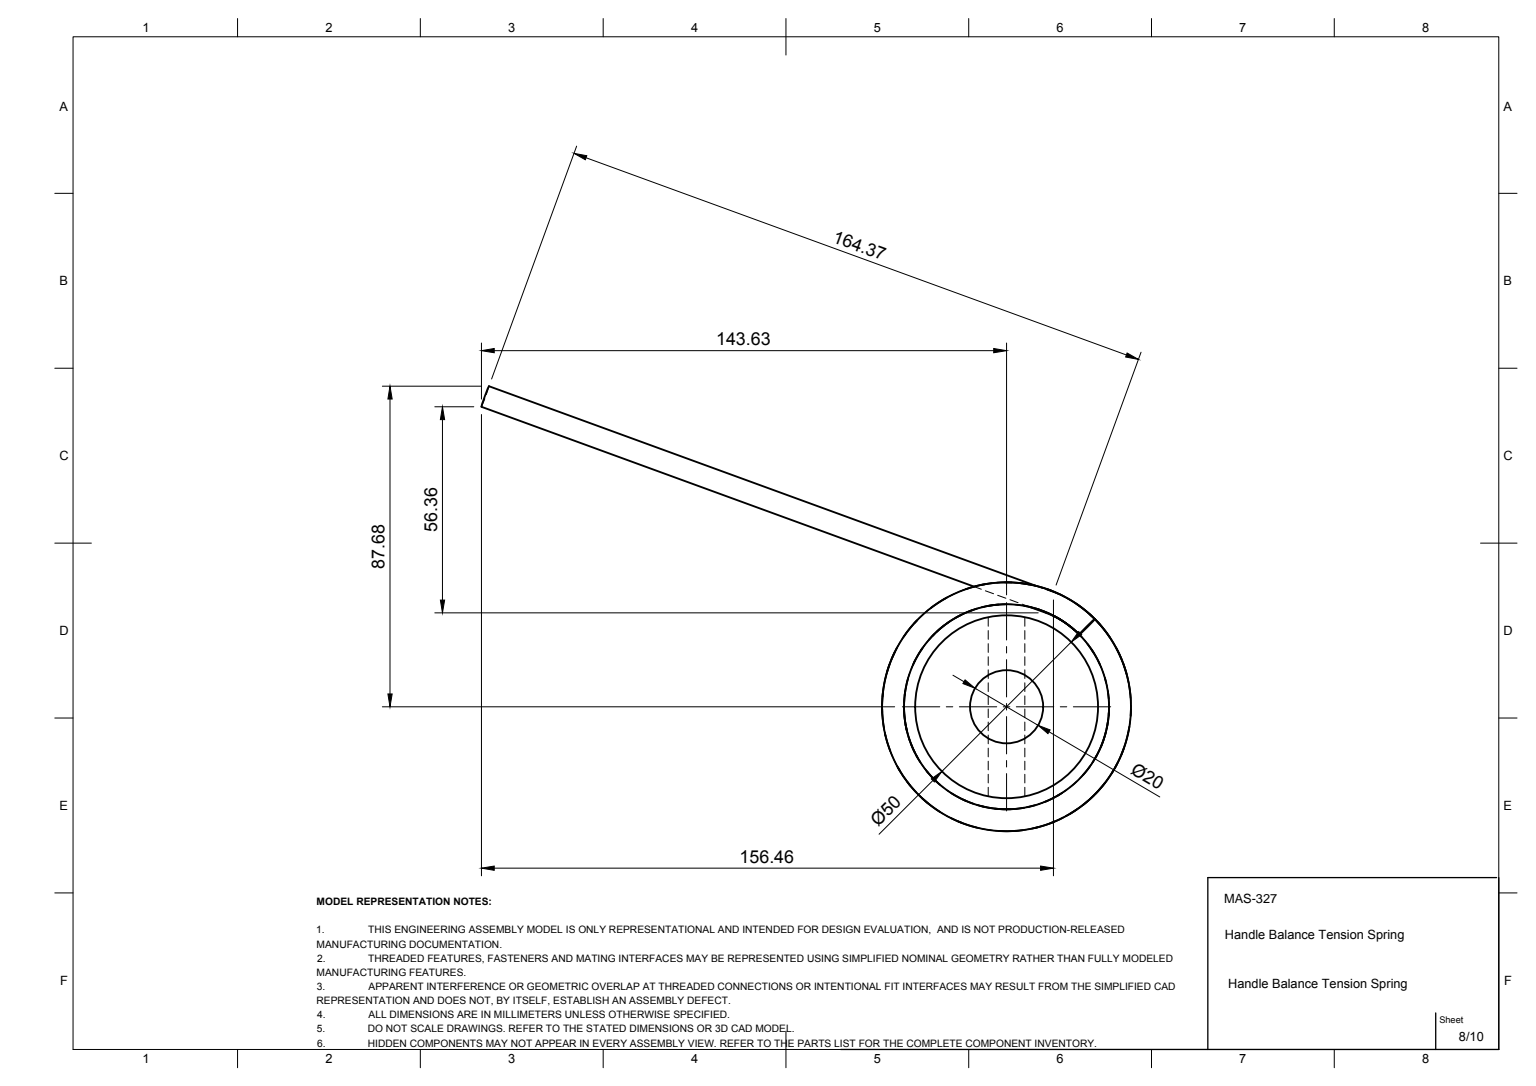
ISO-10303-21;
HEADER;
FILE_DESCRIPTION (('STEP AP214'),
    '1' );
FILE_NAME ('Handle Balance Tension Spring.step',
    '2026-10-06T22:16:42',
    ( '' ),
    ( '' ),
    'SwSTEP 2.0',
    'SolidWorks 2025',
    '' );
FILE_SCHEMA (( 'AUTOMOTIVE_DESIGN' ));
ENDSEC;

DATA;
#5=CARTESIAN_POINT ( 'NONE',  ( 71.26135857449716582, 118.5824631887579272, 4.723566274445706092 ) ) ;
#17=CARTESIAN_POINT ( 'NONE',  ( 22.10153057061799231, 100.9866247252079745, 1.346821830042071566 ) ) ;
#19=CARTESIAN_POINT ( 'NONE',  ( 8.829984022807513711, 121.7968051057545580, 16.14860047415989541 ) ) ;
#30=CARTESIAN_POINT ( 'NONE',  ( 39.19820123626366382, 154.0079489008930693, -4.284297094604833767 ) ) ;
#39=CARTESIAN_POINT ( 'NONE',  ( 43.64334309031418968, 148.0990856179656419, -3.057864931601543823 ) ) ;
#44=CARTESIAN_POINT ( 'NONE',  ( 72.37431012622080573, 137.3510900982057308, 5.986230922049878167 ) ) ;
#53=CARTESIAN_POINT ( 'NONE',  ( 58.35211712195835076, 96.24552883246097679, -7.224606741634919338 ) ) ;
#59=CARTESIAN_POINT ( 'NONE',  ( 77.24268685965694203, 120.2105100216710696, 12.57728155048203433 ) ) ;
#61=CARTESIAN_POINT ( 'NONE',  ( 40.36503175183082703, 91.91162403226272204, -5.481956346182379924 ) ) ;
#81=CARTESIAN_POINT ( 'NONE',  ( 15.47577296012077142, 113.4559151263126040, 0.9141320964044082897 ) ) ;
#87=CARTESIAN_POINT ( 'NONE',  ( 16.50170782505827560, 141.4403336307199197, 3.843654360456687513 ) ) ;
#89=CARTESIAN_POINT ( 'NONE',  ( 29.72792815944318789, 144.7825833525567134, 3.370790685444458479 ) ) ;
#101=CARTESIAN_POINT ( 'NONE',  ( 60.64192606672164487, 149.1585417170215067, -15.56126092485307488 ) ) ;
#109=CARTESIAN_POINT ( 'NONE',  ( 20.88913110926514705, 146.0313881486468119, 3.053432864643822686 ) ) ;
#116=CARTESIAN_POINT ( 'NONE',  ( 14.84555331229717012, 122.4588817147608637, 1.271029365619425144 ) ) ;
#128=CARTESIAN_POINT ( 'NONE',  ( 43.27907770151751521, 148.0257240122537610, -16.07737750751418915 ) ) ;
#140=CARTESIAN_POINT ( 'NONE',  ( 61.83586340360074018, 91.21788411573329824, -1.307985002297802568 ) ) ;
#146=CARTESIAN_POINT ( 'NONE',  ( 9.468627745026951814, 113.0646104733145592, 1.862908727141013854 ) ) ;
#148=CARTESIAN_POINT ( 'NONE',  ( 57.39747520560054284, 144.1616143014069280, -9.486357586414486676 ) ) ;
#154=CARTESIAN_POINT ( 'NONE',  ( 19.03178791447554374, 95.58698510358173905, 9.200771007679692914 ) ) ;
#163=CARTESIAN_POINT ( 'NONE',  ( 16.16443657470430750, 128.5343009702184816, -4.486436360144259616 ) ) ;
#170=DIRECTION ( 'NONE',  ( 1.000000000000000000, 0.000000000000000000, -0.000000000000000000 ) ) ;
#171=CARTESIAN_POINT ( 'NONE',  ( 19.13088699441526686, 95.37848931739559077, 15.19637875606281341 ) ) ;
#173=CARTESIAN_POINT ( 'NONE',  ( 63.17392202723403472, 139.5086487405075673, -1.196242060499778992 ) ) ;
#185=CARTESIAN_POINT ( 'NONE',  ( 14.84555331229717012, 122.4588817147608637, 1.271029365619425144 ) ) ;
#189=CARTESIAN_POINT ( 'NONE',  ( 9.953047844039691228, 128.4882722429139505, 3.367556520687803090 ) ) ;
#190=CARTESIAN_POINT ( 'NONE',  ( 17.20459894546975832, 108.5405110446994001, 1.704077971530460811 ) ) ;
#201=CARTESIAN_POINT ( 'NONE',  ( 44.01981256007524479, 154.0451711359460774, -9.132611258894215212 ) ) ;
#212=CARTESIAN_POINT ( 'NONE',  ( 23.00888394656308122, 147.7027690514567837, -4.855972970016076751 ) ) ;
#219=CARTESIAN_POINT ( 'NONE',  ( 26.43292637418678126, 142.8198486544370098, 2.223537717183381002 ) ) ;
#230=CARTESIAN_POINT ( 'NONE',  ( 33.52710748945926866, 93.34978808121778115, 14.79936193957723312 ) ) ;
#235=CARTESIAN_POINT ( 'NONE',  ( 48.01153233465171866, 95.41220631508043937, 33.88560042642480852 ) ) ;
#245=CARTESIAN_POINT ( 'NONE',  ( 40.94072057685551869, 85.65469043817564909, -0.5939954219232065347 ) ) ;
#251=CARTESIAN_POINT ( 'NONE',  ( 22.46358530849972723, 92.52609567587644790, 8.053519324161520387 ) ) ;
#253=CARTESIAN_POINT ( 'NONE',  ( 60.80507725967250821, 98.03074643439879310, -7.343579217248467295 ) ) ;
#262=CARTESIAN_POINT ( 'NONE',  ( 10.61900875472251649, 108.8314319666055212, -5.279948415675857376 ) ) ;
#272=CARTESIAN_POINT ( 'NONE',  ( 46.66836841558743032, 147.8683539324387368, -2.938892455568735240 ) ) ;
#282=CARTESIAN_POINT ( 'NONE',  ( 68.61421220432494295, 108.2796574941523886, 7.137043325852385323 ) ) ;
#287=ORIENTED_EDGE ( 'NONE', *, *, #12395, .T. ) ;
#301=CARTESIAN_POINT ( 'NONE',  ( 58.57740969237692497, 96.29577388269515836, -1.228997851713355072 ) ) ;
#306=CARTESIAN_POINT ( 'NONE',  ( 15.75986397150585816, 99.18880659646561071, -5.637120474378671808 ) ) ;
#307=CARTESIAN_POINT ( 'NONE',  ( 40.57367117788501787, 91.81261228707245436, 0.5136478283763052932 ) ) ;
#326=CARTESIAN_POINT ( 'NONE',  ( 77.24268685965694203, 120.2105100216710696, 12.57728155048203433 ) ) ;
#332=CARTESIAN_POINT ( 'NONE',  ( 31.11878897118147336, 145.5659923423516773, -4.562434011626001151 ) ) ;
#333=EDGE_CURVE ( 'NONE', #19172, #12901, #10944, .T. ) ;
#334=PRESENTATION_STYLE_ASSIGNMENT (( #15435 ) ) ;
#346=CARTESIAN_POINT ( 'NONE',  ( 42.37836782381873491, 91.71465960395167372, 14.44224817795539373 ) ) ;
#351=CARTESIAN_POINT ( 'NONE',  ( 48.01127559942236900, 95.41215390922535278, 34.53968432338328398 ) ) ;
#353=MANIFOLD_SOLID_BREP ( 'Cut-Extrude12', #11261 ) ;
#359=CARTESIAN_POINT ( 'NONE',  ( 62.34613790317991544, 148.1570561279473850, 11.50573666851796339 ) ) ;
#366=CARTESIAN_POINT ( 'NONE',  ( 8.869018199820361659, 117.4101421016551967, 9.005765870029716069 ) ) ;
#368=CARTESIAN_POINT ( 'NONE',  ( 50.21395344324809429, 147.1711500555979626, 4.203964687196366512 ) ) ;
#374=CARTESIAN_POINT ( 'NONE',  ( 29.43094928344231320, 88.48265962617873015, 0.7917390523231137012 ) ) ;
#382=CARTESIAN_POINT ( 'NONE',  ( 71.13433436327568415, 121.9840874124550965, -8.414894741535439593 ) ) ;
#387=ORIENTED_EDGE ( 'NONE', *, *, #9191, .T. ) ;
#392=CARTESIAN_POINT ( 'NONE',  ( 53.81137604271221164, 145.8702381773545653, 5.351212940250758443 ) ) ;
#395=EDGE_LOOP ( 'NONE', ( #15244, #20080, #9642, #2712 ) ) ;
#409=CARTESIAN_POINT ( 'NONE',  ( 31.65106594408818097, 87.52743543124788062, 20.71565594656193454 ) ) ;
#413=CARTESIAN_POINT ( 'NONE',  ( 21.78317867943344766, 93.15162560046918827, 9.081842247139665147 ) ) ;
#414=CARTESIAN_POINT ( 'NONE',  ( 67.15412698936957270, 134.4792784496449087, 12.06138812558265805 ) ) ;
#423=CARTESIAN_POINT ( 'NONE',  ( 10.57123148683770175, 130.5870355106474108, -10.56118268746274325 ) ) ;
#434=CARTESIAN_POINT ( 'NONE',  ( 68.80033453084351436, 142.5431462587704061, -3.212652714419679700 ) ) ;
#440=CARTESIAN_POINT ( 'NONE',  ( 58.08784223975295902, 95.98046199469133910, 5.794885020722011504 ) ) ;
#450=CARTESIAN_POINT ( 'NONE',  ( 32.23767430054685690, 145.5917660130465379, 17.43780275515692679 ) ) ;
#460=VERTEX_POINT ( 'NONE', #20827 ) ;
#462=CARTESIAN_POINT ( 'NONE',  ( 52.46025766099742071, 152.8098426157893925, 11.14871012209260748 ) ) ;
#467=CARTESIAN_POINT ( 'NONE',  ( 40.02721236285810136, 85.80382532021769748, 0.4343372985580923329 ) ) ;
#469=CARTESIAN_POINT ( 'NONE',  ( 41.25620118372704326, 148.0523446076144580, 3.846850258842608117 ) ) ;
#477=CARTESIAN_POINT ( 'NONE',  ( 20.22230697948889500, 94.36241449208007737, 1.148710122009321211 ) ) ;
#481=CARTESIAN_POINT ( 'NONE',  ( 63.55746018358933469, 147.2895578332197033, -9.446739241148069510 ) ) ;
#494=CARTESIAN_POINT ( 'NONE',  ( 77.13564277734779751, 118.5067815986552375, -14.37074460762677397 ) ) ;
#512=CARTESIAN_POINT ( 'NONE',  ( 26.48090744323847190, 142.7828511622217889, -4.776412194962503577 ) ) ;
#518=CARTESIAN_POINT ( 'NONE',  ( 9.616596702810701558, 112.3753283828585694, -5.161025107254184618 ) ) ;
#519=CARTESIAN_POINT ( 'NONE',  ( 65.09246388851926213, 137.4469437283422906, 4.918530982704383270 ) ) ;
#527=CARTESIAN_POINT ( 'NONE',  ( 42.70556344282044137, 85.75549003223034106, 1.343541076088082376 ) ) ;
#534=CARTESIAN_POINT ( 'NONE',  ( 42.21854335081802390, 85.68333463812091111, 14.36287948008016890 ) ) ;
#540=CARTESIAN_POINT ( 'NONE',  ( 15.53544334784188585, 126.6048195653137469, 15.43757839183889224 ) ) ;
#551=CARTESIAN_POINT ( 'NONE',  ( 63.85057544308668298, 100.9084186779620609, 13.48995955233852229 ) ) ;
#553=CARTESIAN_POINT ( 'NONE',  ( 43.66339603962469340, 144.9006758593374968, 29.24238570022250627 ) ) ;
#556=CARTESIAN_POINT ( 'NONE',  ( 47.56746500088171814, 95.32565373869623215, 32.14446507322556101 ) ) ;
#563=CARTESIAN_POINT ( 'NONE',  ( 26.28242620001017471, 89.94675250444232972, 6.906269859504051922 ) ) ;
#569=CARTESIAN_POINT ( 'NONE',  ( 74.85601106972485752, 107.3429126181175661, -0.9942341299615756745 ) ) ;
#571=CARTESIAN_POINT ( 'NONE',  ( 32.47916914626341622, 146.0660553311768979, 3.489959554161691013 ) ) ;
#580=CARTESIAN_POINT ( 'NONE',  ( 51.60797029699607918, 86.77139250312444574, -6.946567135388369785 ) ) ;
#600=CARTESIAN_POINT ( 'NONE',  ( 19.41497643977705323, 135.2012136132025546, 3.803670830490076149 ) ) ;
#603=CYLINDRICAL_SURFACE ( 'NONE', #15728, 10.00000000000000888 ) ;
#621=CARTESIAN_POINT ( 'NONE',  ( 54.90439719837324617, 94.24896709312837118, 12.93774216356182372 ) ) ;
#627=CARTESIAN_POINT ( 'NONE',  ( 26.87026879109711786, 150.0197496251087728, 11.30891725959585159 ) ) ;
#628=CARTESIAN_POINT ( 'NONE',  ( 68.77576173894735234, 108.4446202281264249, 13.13264940013829296 ) ) ;
#639=CARTESIAN_POINT ( 'NONE',  ( 41.12929731208597417, 154.0090796829547912, -2.227802639778228233 ) ) ;
#648=CARTESIAN_POINT ( 'NONE',  ( 9.231363607564425422, 125.4582397780895633, 16.26765482522027639 ) ) ;
#654=CARTESIAN_POINT ( 'NONE',  ( 46.21245884545565019, 91.80782910428004584, 13.29499484581607582 ) ) ;
#664=CARTESIAN_POINT ( 'NONE',  ( 55.97020510223934764, 144.8627979930266463, -1.553355716038981038 ) ) ;
#676=CARTESIAN_POINT ( 'NONE',  ( 13.60337824163328513, 137.5875211305428252, 8.692014997358331385 ) ) ;
#685=CARTESIAN_POINT ( 'NONE',  ( 70.03002323795641360, 111.8333997399938511, 5.989792257250448060 ) ) ;
#691=CARTESIAN_POINT ( 'NONE',  ( 61.61057083318216598, 91.16763906547615193, -7.303593892219363504 ) ) ;
#703=CARTESIAN_POINT ( 'NONE',  ( 69.71972837475884432, 98.49221204361529658, -7.660766391518695428 ) ) ;
#710=CARTESIAN_POINT ( 'NONE',  ( 43.31828379119179573, 154.0590585871367750, -16.15632009132952973 ) ) ;
#731=CARTESIAN_POINT ( 'NONE',  ( 18.61283035262889385, 105.6058852300018032, 7.580709131559767222 ) ) ;
#738=CARTESIAN_POINT ( 'NONE',  ( 38.34086628137072239, 86.07498427433979771, 8.486398261126511855 ) ) ;
#739=CARTESIAN_POINT ( 'NONE',  ( 16.97565887011968400, 109.0741130153051444, 8.727962422049884594 ) ) ;
#746=CARTESIAN_POINT ( 'NONE',  ( 31.96084264191244273, 87.59053552682176758, 1.700516636338098797 ) ) ;
#754=CARTESIAN_POINT ( 'NONE',  ( 29.59780345622613851, 88.32329120701308511, 6.787350155335245994 ) ) ;
#760=CARTESIAN_POINT ( 'NONE',  ( 70.16915148685765757, 112.0176666281686977, 11.98539833154344691 ) ) ;
#774=CARTESIAN_POINT ( 'NONE',  ( 32.71008791447857789, 146.0719641954536883, -2.505641559509553140 ) ) ;
#776=CARTESIAN_POINT ( 'NONE',  ( 45.52055293674428071, 144.7823678009017954, 38.54804764342389944 ) ) ;
#781=DIRECTION ( 'NONE',  ( 0.9387810623359076345, 0.3426822732243071656, 0.03548206049944094970 ) ) ;
#785=CARTESIAN_POINT ( 'NONE',  ( 51.15470623622070434, 86.57325545146775880, 6.072769092256255163 ) ) ;
#793=CARTESIAN_POINT ( 'NONE',  ( 67.98812442775457043, 106.8157236907426153, -0.7957547315468347371 ) ) ;
#800=CARTESIAN_POINT ( 'NONE',  ( 75.16956835342354282, 131.6452004531123805, 5.196376467030073165 ) ) ;
#809=CARTESIAN_POINT ( 'NONE',  ( 75.85495621331871519, 129.5603373922052697, -8.732165470513974626 ) ) ;
#815=CARTESIAN_POINT ( 'NONE',  ( 15.58850788081759475, 140.2644050767460442, -10.20415289822252980 ) ) ;
#836=CARTESIAN_POINT ( 'NONE',  ( 29.49905557571407044, 144.7517438296894738, 9.366394860000250233 ) ) ;
#842=CARTESIAN_POINT ( 'NONE',  ( 18.20936163119166196, 143.5026679720446907, 2.934308097026923967 ) ) ;
#843=CARTESIAN_POINT ( 'NONE',  ( 65.44800906011916197, 136.9904114405718758, 11.94221925691594777 ) ) ;
#844=CARTESIAN_POINT ( 'NONE',  ( 20.98687704487253569, 141.7792436784441747, -11.00219731500033049 ) ) ;
#853=CARTESIAN_POINT ( 'NONE',  ( 9.783399875253829592, 127.8057224500684015, -3.656374068424393275 ) ) ;
#855=CARTESIAN_POINT ( 'NONE',  ( 70.26356658872128946, 140.6255928306487704, 11.86290872716119615 ) ) ;
#861=CARTESIAN_POINT ( 'NONE',  ( 10.61292492956169475, 108.6005711365770026, 0.7156557588857267449 ) ) ;
#869=CARTESIAN_POINT ( 'NONE',  ( 43.17520790721623314, 91.62706341066298421, 13.41396976009479403 ) ) ;
#878=CARTESIAN_POINT ( 'NONE',  ( 14.99696000743431235, 117.4761687382565327, -3.934212988072375516 ) ) ;
#891=CARTESIAN_POINT ( 'NONE',  ( 54.37136329154349568, 152.2862128563062072, 3.215626235130811583 ) ) ;
#898=CARTESIAN_POINT ( 'NONE',  ( 39.35338560254503903, 91.94623120232463975, 14.56122079753911081 ) ) ;
#904=CARTESIAN_POINT ( 'NONE',  ( 62.84376099716368458, 92.00366499689042143, 13.64888190966157566 ) ) ;
#915=CARTESIAN_POINT ( 'NONE',  ( 15.75986397150585816, 99.18880659646561071, -5.637120474378671808 ) ) ;
#925=ORIENTED_EDGE ( 'NONE', *, *, #19064, .F. ) ;
#940=CARTESIAN_POINT ( 'NONE',  ( 40.78231060393920870, 91.71360054188218669, 6.509252002934985626 ) ) ;
#946=CARTESIAN_POINT ( 'NONE',  ( 57.14511974427749408, 88.72838517433189054, 6.862995836283489304 ) ) ;
#948=CARTESIAN_POINT ( 'NONE',  ( 16.70103016558074316, 129.9804388327498827, 16.57432765154378629 ) ) ;
#949=CARTESIAN_POINT ( 'NONE',  ( 26.28921445626723852, 149.7786157371718616, -3.732453678475698311 ) ) ;
#959=CARTESIAN_POINT ( 'NONE',  ( 47.07528247981900904, 85.99676402675389397, -5.799316066731655006 ) ) ;
#961=CARTESIAN_POINT ( 'NONE',  ( 31.47436479266152531, 87.67613096727390598, 14.72005176623422606 ) ) ;
#968=CARTESIAN_POINT ( 'NONE',  ( 75.01029411920679024, 107.5147569559006655, 5.001370044594233732 ) ) ;
#974=CARTESIAN_POINT ( 'NONE',  ( 70.54646159239726444, 126.3605644061445901, 18.41388650843374464 ) ) ;
#982=ORIENTED_EDGE ( 'NONE', *, *, #5579, .F. ) ;
#987=CARTESIAN_POINT ( 'NONE',  ( 68.32201692705490359, 132.1587870917933003, -0.8393580998851425390 ) ) ;
#990=CARTESIAN_POINT ( 'NONE',  ( 46.98099381664906815, 144.5901365555967004, 37.25520735466820810 ) ) ;
#996=CARTESIAN_POINT ( 'NONE',  ( 23.17700876947760591, 147.8092992330439586, -3.851376987104358829 ) ) ;
#1003=CARTESIAN_POINT ( 'NONE',  ( 73.37616494982036386, 135.8902282719419077, 4.049127002338204662 ) ) ;
#1012=CARTESIAN_POINT ( 'NONE',  ( 33.52710748945926866, 93.34978808121778115, 14.79936193957723312 ) ) ;
#1019=CARTESIAN_POINT ( 'NONE',  ( 71.03835150376274044, 100.2492380157770526, 6.267546321443639989 ) ) ;
#1028=CARTESIAN_POINT ( 'NONE',  ( 57.94507594753278568, 150.7106492751291569, -2.660852849641732298 ) ) ;
#1036=ADVANCED_FACE ( 'NONE', ( #2390 ), #7256, .F. ) ;
#1052=CARTESIAN_POINT ( 'NONE',  ( 34.49559591455799534, 146.8750064778945728, 2.580435534661669195 ) ) ;
#1055=DIRECTION ( 'NONE',  ( -1.000000000000000000, 0.000000000000000000, 0.000000000000000000 ) ) ;
#1058=CARTESIAN_POINT ( 'NONE',  ( 54.54805624998882507, 152.1374805055981199, -2.779977617235711129 ) ) ;
#1060=CARTESIAN_POINT ( 'NONE',  ( 43.85786119575681852, 148.0137586191354444, -9.053472026759274982 ) ) ;
#1062=CARTESIAN_POINT ( 'NONE',  ( 23.67598417054553295, 91.65793073385727041, -5.994147020910363999 ) ) ;
#1072=CARTESIAN_POINT ( 'NONE',  ( 8.922311181598237440, 122.0085103898528018, 10.15299703236346573 ) ) ;
#1075=CARTESIAN_POINT ( 'NONE',  ( 72.33162239183086228, 137.5781058455011703, 11.98183203572534872 ) ) ;
#1080=CARTESIAN_POINT ( 'NONE',  ( 43.59077634914400079, 154.2158251336064723, 2.858602931426994953 ) ) ;
#1086=CARTESIAN_POINT ( 'NONE',  ( 58.78870511939484800, 143.3781512503299780, 17.58070913143554748 ) ) ;
#1091=PLANE ( 'NONE',  #19799 ) ;
#1097=CARTESIAN_POINT ( 'NONE',  ( 37.89917375590665927, 147.5588116854153498, -9.291614562240097186 ) ) ;
#1098=CARTESIAN_POINT ( 'NONE',  ( 43.66945230930459587, 144.9005013971865594, 39.17809732472422013 ) ) ;
#1104=CARTESIAN_POINT ( 'NONE',  ( 23.67598417054553295, 91.65793073385727041, -5.994147020910363999 ) ) ;
#1112=CARTESIAN_POINT ( 'NONE',  ( 41.39294982251618649, 154.1830292177732531, 16.78735015533800734 ) ) ;
#1119=CARTESIAN_POINT ( 'NONE',  ( 25.64412274706724304, 97.69032544021251852, 15.15625305551708202 ) ) ;
#1127=CARTESIAN_POINT ( 'NONE',  ( 40.90832812944997698, 154.0758954209757121, 3.767805038447253452 ) ) ;
#1128=CARTESIAN_POINT ( 'NONE',  ( 40.50225576765475921, 95.03178743630938641, 38.54804764342390655 ) ) ;
#1136=CARTESIAN_POINT ( 'NONE',  ( 69.83118287335672392, 141.1824132108841638, 4.838974892866481525 ) ) ;
#1161=CARTESIAN_POINT ( 'NONE',  ( 39.55749537675153960, 91.83829536962669238, 20.55682687220188143 ) ) ;
#1167=CARTESIAN_POINT ( 'NONE',  ( 47.47886434171987702, 153.8471147930492862, -3.017879606865911502 ) ) ;
#1168=CARTESIAN_POINT ( 'NONE',  ( 68.06566224877710169, 132.6756899087416457, -7.863043133634088910 ) ) ;
#1176=CARTESIAN_POINT ( 'NONE',  ( 56.11190468687431832, 151.4478768383145280, 5.272225788895710252 ) ) ;
#1181=EDGE_CURVE ( 'NONE', #11596, #5848, #13724, .T. ) ;
#1185=CARTESIAN_POINT ( 'NONE',  ( 9.585575214713108139, 112.1464265272871188, 0.8345760063739874335 ) ) ;
#1191=CARTESIAN_POINT ( 'NONE',  ( 66.16974147772015158, 135.9983230778657344, -9.010293137571032673 ) ) ;
#1200=CARTESIAN_POINT ( 'NONE',  ( 48.12388674207330297, 92.25590008057444891, 8.208355790051324874 ) ) ;
#1204=CARTESIAN_POINT ( 'NONE',  ( 47.85046472749336743, 144.4343633168767269, 32.91075569967801329 ) ) ;
#1220=CARTESIAN_POINT ( 'NONE',  ( 10.76517401744387215, 131.6399553617083029, 15.47769843104460463 ) ) ;
#1223=CARTESIAN_POINT ( 'NONE',  ( 9.504183449854689769, 113.2927979568517571, -4.132695447411913747 ) ) ;
#1226=CARTESIAN_POINT ( 'NONE',  ( 14.85320491933239317, 121.4429315054255909, 16.22795414098078126 ) ) ;
#1230=CARTESIAN_POINT ( 'NONE',  ( 15.00983914341701997, 123.2415857317943448, 2.299110145932334426 ) ) ;
#1232=CARTESIAN_POINT ( 'NONE',  ( 65.27013532398795803, 145.9152199903044504, 11.62486143609835310 ) ) ;
#1243=CARTESIAN_POINT ( 'NONE',  ( 26.90790578767411390, 150.1165885900122987, 3.291480155758420345 ) ) ;
#1269=CARTESIAN_POINT ( 'NONE',  ( 69.69253243162556544, 129.2828754355126648, 18.29472124897268159 ) ) ;
#1276=CARTESIAN_POINT ( 'NONE',  ( 63.41425016244589585, 92.41789933959738335, 6.624947895572852019 ) ) ;
#1277=CARTESIAN_POINT ( 'NONE',  ( 69.05514009256096131, 130.5101840208823205, -14.76775785107876082 ) ) ;
#1294=CARTESIAN_POINT ( 'NONE',  ( 26.67903320394502131, 150.0857490671680807, 9.287084330314211655 ) ) ;
#1301=CARTESIAN_POINT ( 'NONE',  ( 59.92122946415073415, 142.4742691614619332, -9.367183195626855863 ) ) ;
#1311=CARTESIAN_POINT ( 'NONE',  ( 33.24893159794274311, 146.2783277815063059, 4.518043653832040540 ) ) ;
#1321=CARTESIAN_POINT ( 'NONE',  ( 46.60148787037231699, 85.86292235506145687, 7.220022382731924537 ) ) ;
#1328=CARTESIAN_POINT ( 'NONE',  ( 63.06653971011325410, 92.06373373134326243, 19.64449301269484849 ) ) ;
#1329=CIRCLE ( 'NONE', #8736, 24.99999999999999289 ) ;
#1332=CARTESIAN_POINT ( 'NONE',  ( 15.69291839309778958, 99.40984958608130739, -11.63272432674803802 ) ) ;
#1336=CARTESIAN_POINT ( 'NONE',  ( 44.86974823489592978, 148.0457227541334362, 10.98970740178311090 ) ) ;
#1341=CARTESIAN_POINT ( 'NONE',  ( 17.20459894546975832, 108.5405110446994001, 1.704077971530460811 ) ) ;
#1345=CARTESIAN_POINT ( 'NONE',  ( 41.71169011715027608, 94.93878194014966709, 29.37128083581765381 ) ) ;
#1355=CARTESIAN_POINT ( 'NONE',  ( 26.13368487350976110, 90.12329638092472806, 0.9106621812756837686 ) ) ;
#1379=CARTESIAN_POINT ( 'NONE',  ( 26.70363248220801466, 142.8423586596025245, -10.77201286955609127 ) ) ;
#1385=CARTESIAN_POINT ( 'NONE',  ( 16.30372524420941716, 141.3216567370616019, 9.839263250375132941 ) ) ;
#1388=CARTESIAN_POINT ( 'NONE',  ( 40.25662930883660806, 147.8909896968035014, -16.19631701608006580 ) ) ;
#1405=CARTESIAN_POINT ( 'NONE',  ( 62.21295035458982881, 148.3457431455455549, 17.50134052088148096 ) ) ;
#1412=CARTESIAN_POINT ( 'NONE',  ( 24.63684302007652249, 148.6959638282970957, 4.200683933265449532 ) ) ;
#1413=CARTESIAN_POINT ( 'NONE',  ( 69.04633063039527485, 130.7408809369782716, -8.772150750671475095 ) ) ;
#1423=CARTESIAN_POINT ( 'NONE',  ( 15.29689364450883815, 124.6620785063593786, 10.35143954082134954 ) ) ;
#1433=CARTESIAN_POINT ( 'NONE',  ( 67.39040179371399120, 143.9404232637865562, 4.720051584306741432 ) ) ;
#1442=CARTESIAN_POINT ( 'NONE',  ( 21.21153947156776809, 146.4065673692475400, 16.07276909216647454 ) ) ;
#1446=CARTESIAN_POINT ( 'NONE',  ( 13.64837572802379562, 102.4646860582014796, -11.51360178106338594 ) ) ;
#1454=CARTESIAN_POINT ( 'NONE',  ( 63.07923660420441792, 139.7192868340247571, 4.799362114056002326 ) ) ;
#1466=CARTESIAN_POINT ( 'NONE',  ( 40.90832812944997698, 154.0758954209757121, 3.767805038447253452 ) ) ;
#1472=CARTESIAN_POINT ( 'NONE',  ( 61.61057083318216598, 91.16763906547615193, -7.303593892219363504 ) ) ;
#1492=CARTESIAN_POINT ( 'NONE',  ( 19.04663372520828801, 134.9227921665808765, 15.79488502079956547 ) ) ;
#1498=CARTESIAN_POINT ( 'NONE',  ( 55.94180145820917716, 151.6039095241057453, 11.26783467880839140 ) ) ;
#1499=CARTESIAN_POINT ( 'NONE',  ( 47.44511438772692458, 147.6747606579048409, -1.910614883896327054 ) ) ;
#1517=CARTESIAN_POINT ( 'NONE',  ( 70.82039710638956365, 99.80338443054456832, 19.28708432993385102 ) ) ;
#1522=CARTESIAN_POINT ( 'NONE',  ( 59.50342836137831171, 89.99885106877826502, 7.772197353298202493 ) ) ;
#1523=CARTESIAN_POINT ( 'NONE',  ( 55.20039838223064521, 94.47806301326188816, -0.08174959847185196693 ) ) ;
#1532=CARTESIAN_POINT ( 'NONE',  ( 71.12409474721032154, 120.5409021055102841, -0.3630727742139398528 ) ) ;
#1544=CARTESIAN_POINT ( 'NONE',  ( 47.30009524607925897, 85.94413156685014599, 0.1962900075584997628 ) ) ;
#1551=CARTESIAN_POINT ( 'NONE',  ( 22.89857099655110062, 139.5608133708311982, -4.966967973427480310 ) ) ;
#1554=CARTESIAN_POINT ( 'NONE',  ( 17.52322149637394233, 97.17389352242535949, -4.727774211004094340 ) ) ;
#1564=CARTESIAN_POINT ( 'NONE',  ( 25.21830160582964453, 141.7844325674071229, 10.15653385063274428 ) ) ;
#1567=CARTESIAN_POINT ( 'NONE',  ( 15.97061701817242785, 140.8453463817331794, 16.82122940411608170 ) ) ;
#1576=CARTESIAN_POINT ( 'NONE',  ( 53.71239221804358976, 87.38980250447106357, 6.982120393166105998 ) ) ;
#1583=CARTESIAN_POINT ( 'NONE',  ( 40.73010619540765020, 85.74955863377461185, -6.589596535617429751 ) ) ;
#1585=CARTESIAN_POINT ( 'NONE',  ( 26.70363248220801466, 142.8423586596025245, -10.77201286955609127 ) ) ;
#1589=CARTESIAN_POINT ( 'NONE',  ( 62.62098228421420032, 91.94359626243755201, 7.653270806628301948 ) ) ;
#1597=CARTESIAN_POINT ( 'NONE',  ( 57.03263806925237844, 95.34629841206742640, 19.84245794357962822 ) ) ;
#1604=CARTESIAN_POINT ( 'NONE',  ( 76.40658810299491677, 127.4365358892444959, 12.33923360994393903 ) ) ;
#1605=CARTESIAN_POINT ( 'NONE',  ( 54.97053026609068382, 94.45704024927961484, -6.077358488390353308 ) ) ;
#1623=CARTESIAN_POINT ( 'NONE',  ( 63.63589212299756070, 92.48244826560708987, 12.62055557379543203 ) ) ;
#1628=CARTESIAN_POINT ( 'NONE',  ( 67.48508721674359379, 143.7297851702464015, -1.275552590249036777 ) ) ;
#1629=CARTESIAN_POINT ( 'NONE',  ( 49.55020742284296631, 92.47612394764220767, 0.1565338505643876776 ) ) ;
#1641=CARTESIAN_POINT ( 'NONE',  ( 54.44380493464903736, 94.21656919670213881, 0.9465279732350617703 ) ) ;
#1653=CARTESIAN_POINT ( 'NONE',  ( 73.72238702602700755, 135.0318370961144296, 5.077453337991364002 ) ) ;
#1659=CARTESIAN_POINT ( 'NONE',  ( 66.44170838958859804, 135.7440291252205213, 4.009006963233090026 ) ) ;
#1673=CARTESIAN_POINT ( 'NONE',  ( 70.94289844336020678, 123.7826807253454575, 5.513563639855703080 ) ) ;
#1687=CARTESIAN_POINT ( 'NONE',  ( 75.87089013534350102, 129.7906142932847331, -2.736556584054479657 ) ) ;
#1694=CARTESIAN_POINT ( 'NONE',  ( 69.71972837475884432, 98.49221204361529658, -7.660766391518695428 ) ) ;
#1698=CARTESIAN_POINT ( 'NONE',  ( 16.33471683235446292, 110.7640000046674089, -5.200637885961103102 ) ) ;
#1704=CARTESIAN_POINT ( 'NONE',  ( 71.86557814238962294, 101.4853659568252766, -7.779689512009451136 ) ) ;
#1712=CARTESIAN_POINT ( 'NONE',  ( 71.19430100617981338, 118.9508470517051535, -8.295922056425867552 ) ) ;
#1721=CARTESIAN_POINT ( 'NONE',  ( 9.231363607564425422, 125.4582397780895633, 16.26765482522027639 ) ) ;
#1723=CARTESIAN_POINT ( 'NONE',  ( 24.98902006629997175, 141.4916631675600343, -2.862956674147950409 ) ) ;
#1736=CARTESIAN_POINT ( 'NONE',  ( 71.19881468907274780, 122.2058620619881566, -2.419290889312981641 ) ) ;
#1742=CARTESIAN_POINT ( 'NONE',  ( 42.70556344282044137, 85.75549003223034106, 1.343541076088082376 ) ) ;
#1743=CARTESIAN_POINT ( 'NONE',  ( 62.66823040046688931, 140.1266048904901993, -2.224326160187301227 ) ) ;
#1751=DIRECTION ( 'NONE',  ( 0.000000000000000000, 0.000000000000000000, 1.000000000000000000 ) ) ;
#1754=CARTESIAN_POINT ( 'NONE',  ( 29.68407903333335085, 144.6596297928226988, 11.33750686376150085 ) ) ;
#1763=CARTESIAN_POINT ( 'NONE',  ( 9.468627745026951814, 113.0646104733145592, 1.862908727141013854 ) ) ;
#1770=CARTESIAN_POINT ( 'NONE',  ( 18.91286941000743838, 105.1068529970173699, 0.5568269029779387980 ) ) ;
#1783=CARTESIAN_POINT ( 'NONE',  ( 53.64127281404707048, 146.0262708631457542, 11.34682183016344403 ) ) ;
#1792=CARTESIAN_POINT ( 'NONE',  ( 39.03606557573836255, 144.5896687849443651, 31.16068397573688387 ) ) ;
#1795=ORIENTED_EDGE ( 'NONE', *, *, #13768, .T. ) ;
#1798=CARTESIAN_POINT ( 'NONE',  ( 64.81014823317600815, 93.40725510594978687, -1.427111354441281899 ) ) ;
#1803=CARTESIAN_POINT ( 'NONE',  ( 73.32203938827501588, 103.9946350594383517, -0.8753108214479579097 ) ) ;
#1805=CARTESIAN_POINT ( 'NONE',  ( 49.02192908010439254, 147.4586317741252799, -9.843465619175002956 ) ) ;
#1811=CARTESIAN_POINT ( 'NONE',  ( 42.00398509169406935, 85.76881261499585207, 8.367275628961508005 ) ) ;
#1820=CARTESIAN_POINT ( 'NONE',  ( 68.03731475862628031, 132.9047928164914367, -1.867435455408581912 ) ) ;
#1827=CARTESIAN_POINT ( 'NONE',  ( 28.07864021081662287, 89.10199518432737875, 14.83897397183228861 ) ) ;
#1829=CARTESIAN_POINT ( 'NONE',  ( 70.19721620597543676, 127.0927327670264475, -7.624900598222268400 ) ) ;
#1846=CARTESIAN_POINT ( 'NONE',  ( 50.34320592624661828, 92.59351467088818310, -0.8717445255428065698 ) ) ;
#1850=CARTESIAN_POINT ( 'NONE',  ( 20.25093610150840107, 136.5556286039603435, -4.129180435126924564 ) ) ;
#1853=VERTEX_POINT ( 'NONE', #14705 ) ;
#1854=DIRECTION ( 'NONE',  ( 0.000000000000000000, 0.000000000000000000, 1.000000000000000000 ) ) ;
#1860=CARTESIAN_POINT ( 'NONE',  ( 39.64555921537804295, 153.8934876517313342, -16.27550955686750456 ) ) ;
#1869=CARTESIAN_POINT ( 'NONE',  ( 23.42018083028975184, 147.9700754799198705, 17.16443675223517573 ) ) ;
#1875=CARTESIAN_POINT ( 'NONE',  ( 70.23874406963963679, 127.5525917602273012, 4.366313592093098883 ) ) ;
#1885=CARTESIAN_POINT ( 'NONE',  ( 17.81206540393426252, 132.5069038242342003, 16.68302557436956945 ) ) ;
#1891=CARTESIAN_POINT ( 'NONE',  ( 41.71002329038685730, 144.8752540357612020, 29.37189892749851694 ) ) ;
#1896=CARTESIAN_POINT ( 'NONE',  ( 42.21854335081802390, 85.68333463812091111, 14.36287948008016890 ) ) ;
#1901=CARTESIAN_POINT ( 'NONE',  ( 20.98687704487253569, 141.7792436784441747, -11.00219731500033049 ) ) ;
#1903=CARTESIAN_POINT ( 'NONE',  ( 46.60148787037231699, 85.86292235506145687, 7.220022382731924537 ) ) ;
#1911=CARTESIAN_POINT ( 'NONE',  ( 9.468627745026951814, 113.0646104733145592, 1.862908727141013854 ) ) ;
#1921=CARTESIAN_POINT ( 'NONE',  ( 55.29376081731632553, 145.2908078538121401, -2.581636314160848489 ) ) ;
#1927=ORIENTED_EDGE ( 'NONE', *, *, #17355, .T. ) ;
#1932=CARTESIAN_POINT ( 'NONE',  ( 50.52618006956270591, 153.2232370340747138, -15.91843667049845834 ) ) ;
#1944=CARTESIAN_POINT ( 'NONE',  ( 18.86674891209848326, 143.9013856721611546, -11.04182128657428485 ) ) ;
#1951=CARTESIAN_POINT ( 'NONE',  ( 16.02160000510927418, 128.3529272436884128, 1.509170735004851549 ) ) ;
#1955=CARTESIAN_POINT ( 'NONE',  ( 30.08091612619420729, 88.20954595054467973, -6.232194961517499188 ) ) ;
#1956=CARTESIAN_POINT ( 'NONE',  ( 14.81332417359726783, 119.6334487847019403, -4.843746996953559147 ) ) ;
#1967=CARTESIAN_POINT ( 'NONE',  ( 20.91795382191701336, 137.2581800298614212, 10.90446256675174297 ) ) ;
#1977=CARTESIAN_POINT ( 'NONE',  ( 45.29500579500201951, 154.0643053174194961, 10.91066218119221709 ) ) ;
#1983=CARTESIAN_POINT ( 'NONE',  ( 14.73513546934961482, 119.4163655414939740, 1.151864106104608432 ) ) ;
#1984=SURFACE_SIDE_STYLE ('',( #20397 ) ) ;
#1996=CARTESIAN_POINT ( 'NONE',  ( 31.57890723221301599, 145.5991046824261446, -16.55366158474257432 ) ) ;
#2002=CARTESIAN_POINT ( 'NONE',  ( 44.62651314315545648, 94.95745790197152303, 38.95396702123348831 ) ) ;
#2007=ORIENTED_EDGE ( 'NONE', *, *, #6812, .F. ) ;
#2010=CARTESIAN_POINT ( 'NONE',  ( 32.07966263401961982, 152.4337125855422528, -4.522337938825778281 ) ) ;
#2017=CARTESIAN_POINT ( 'NONE',  ( 17.14282613681034917, 97.48634091255654255, 8.291567264837656381 ) ) ;
#2019=CARTESIAN_POINT ( 'NONE',  ( 15.50679444821833819, 113.6848169819070193, -5.081469017220888063 ) ) ;
#2027=CARTESIAN_POINT ( 'NONE',  ( 40.73010619540765020, 85.74955863377461185, -6.589596535617429751 ) ) ;
#2034=CARTESIAN_POINT ( 'NONE',  ( 41.15066532084431827, 91.76888749123396849, -6.510040445920065366 ) ) ;
#2044=CARTESIAN_POINT ( 'NONE',  ( 21.19424684193554143, 137.6478987072957807, 3.922641511544080917 ) ) ;
#2064=CARTESIAN_POINT ( 'NONE',  ( 29.98029990418277180, 151.1550010424932111, 23.43402463578956585 ) ) ;
#2068=CARTESIAN_POINT ( 'NONE',  ( 64.59149290518072917, 93.33317027722591774, -7.422718449586769296 ) ) ;
#2070=CARTESIAN_POINT ( 'NONE',  ( 61.33076419740685736, 141.3451534613812441, 11.70407797152743079 ) ) ;
#2078=CARTESIAN_POINT ( 'NONE',  ( 73.43285993012185031, 135.4320224564883688, -7.942088354107054826 ) ) ;
#2087=CARTESIAN_POINT ( 'NONE',  ( 14.48810111090402941, 100.9784058478479523, 15.43442115621699529 ) ) ;
#2093=CARTESIAN_POINT ( 'NONE',  ( 41.03523200113699687, 148.1191603456353789, 9.842457937073838536 ) ) ;
#2101=CARTESIAN_POINT ( 'NONE',  ( 58.92189266798492042, 143.1894642327317513, 11.58510527907202992 ) ) ;
#2103=CARTESIAN_POINT ( 'NONE',  ( 45.22414464412956647, 144.8093836198929694, 29.72396354041403299 ) ) ;
#2115=CARTESIAN_POINT ( 'NONE',  ( 12.43312601512511151, 135.2277911470865490, 16.60371454366222466 ) ) ;
#2121=CARTESIAN_POINT ( 'NONE',  ( 30.24639091383375700, 151.6717570033048048, 3.410403464249057492 ) ) ;
#2123=CARTESIAN_POINT ( 'NONE',  ( 16.97565887011968400, 109.0741130153051444, 8.727962422049884594 ) ) ;
#2130=CARTESIAN_POINT ( 'NONE',  ( 17.73005198514846725, 142.9879744078657779, -4.089424278207452801 ) ) ;
#2132=CARTESIAN_POINT ( 'NONE',  ( 20.22230697948889500, 94.36241449208007737, 1.148710122009321211 ) ) ;
#2137=CARTESIAN_POINT ( 'NONE',  ( 40.73010619540765020, 85.74955863377461185, -6.589596535617429751 ) ) ;
#2149=CARTESIAN_POINT ( 'NONE',  ( 75.83902229129397199, 129.3300604911257778, -14.72777435697347137 ) ) ;
#2165=CARTESIAN_POINT ( 'NONE',  ( 70.48772827241290884, 113.2068808858050630, -2.062176545857650201 ) ) ;
#2169=CARTESIAN_POINT ( 'NONE',  ( 30.38027039762175718, 151.3010018550503446, 11.44158087452429129 ) ) ;
#2170=CARTESIAN_POINT ( 'NONE',  ( 63.07923660420441792, 139.7192868340247571, 4.799362114056002326 ) ) ;
#2180=CARTESIAN_POINT ( 'NONE',  ( 29.91082003397629663, 88.36561978549612206, -12.22780263974880022 ) ) ;
#2193=CARTESIAN_POINT ( 'NONE',  ( 62.34613790317991544, 148.1570561279473850, 11.50573666851796339 ) ) ;
#2200=CARTESIAN_POINT ( 'NONE',  ( 17.32321720400341292, 131.7349665092470730, 8.652027877775747555 ) ) ;
#2210=CARTESIAN_POINT ( 'NONE',  ( 51.29519266978688563, 92.95216133272363379, 14.08499220319455780 ) ) ;
#2216=CARTESIAN_POINT ( 'NONE',  ( 43.01140435219951286, 94.90707761860558378, 39.21067981925356349 ) ) ;
#2223=CARTESIAN_POINT ( 'NONE',  ( 61.24245875951225315, 90.83725678726602837, 5.715745788549559059 ) ) ;
#2228=CARTESIAN_POINT ( 'NONE',  ( 29.43094928344231320, 88.48265962617873015, 0.7917390523231137012 ) ) ;
#2231=CARTESIAN_POINT ( 'NONE',  ( 69.25106277675128297, 109.5764507715396832, -0.9149236002526208722 ) ) ;
#2237=CARTESIAN_POINT ( 'NONE',  ( 76.04618105687035268, 128.8835079444423286, -1.708432735116285350 ) ) ;
#2247=CARTESIAN_POINT ( 'NONE',  ( 76.04618105687035268, 128.8835079444423286, -1.708432735116285350 ) ) ;
#2248=FACE_OUTER_BOUND ( 'NONE', #9607, .T. ) ;
#2253=CARTESIAN_POINT ( 'NONE',  ( 15.21076168709227616, 115.6846582791190201, 9.994193321846964295 ) ) ;
#2269=CARTESIAN_POINT ( 'NONE',  ( 50.02529374262071826, 147.3041493969045064, 10.19957357710909207 ) ) ;
#2273=CARTESIAN_POINT ( 'NONE',  ( 9.248697603757472407, 114.7582530722838356, 9.914954709382596931 ) ) ;
#2274=CARTESIAN_POINT ( 'NONE',  ( 25.64412274706724304, 97.69032544021251852, 15.15625305551708202 ) ) ;
#2283=CARTESIAN_POINT ( 'NONE',  ( 46.37776046713125311, 85.92026137128108587, 1.224418530371263580 ) ) ;
#2286=CARTESIAN_POINT ( 'NONE',  ( 26.66797635711824199, 149.9459070286683868, 17.30505193804556185 ) ) ;
#2292=CARTESIAN_POINT ( 'NONE',  ( 9.976645104453018220, 110.9295780357170571, 15.79146183154218619 ) ) ;
#2298=CARTESIAN_POINT ( 'NONE',  ( 47.04142330690687857, 147.8988775214238842, 10.08059930640748902 ) ) ;
#2311=CARTESIAN_POINT ( 'NONE',  ( 24.98902006629997175, 141.4916631675600343, -2.862956674147950409 ) ) ;
#2313=CARTESIAN_POINT ( 'NONE',  ( 46.31438439993811329, 144.6890179153603242, 30.44285285587857715 ) ) ;
#2318=CARTESIAN_POINT ( 'NONE',  ( 45.51857396895002239, 95.03161353365992170, 38.54896506029344749 ) ) ;
#2322=ADVANCED_FACE ( 'NONE', ( #14541 ), #13705, .T. ) ;
#2325=CARTESIAN_POINT ( 'NONE',  ( 69.47322557110069852, 98.06143112153284846, 5.358778726746561638 ) ) ;
#2333=CARTESIAN_POINT ( 'NONE',  ( 66.10898071834657230, 103.7292514542787245, 6.347102411281516865 ) ) ;
#2341=CARTESIAN_POINT ( 'NONE',  ( 77.19215121279506775, 118.0176990621192203, -1.351406188750652992 ) ) ;
#2354=CARTESIAN_POINT ( 'NONE',  ( 60.49690154327523572, 149.3382625450468311, -9.565656633516235630 ) ) ;
#2360=CARTESIAN_POINT ( 'NONE',  ( 32.54106024366770811, 152.4163610972421452, -16.51355214031335805 ) ) ;
#2381=CARTESIAN_POINT ( 'NONE',  ( 68.16012629694054681, 106.9699110742356396, 5.199846382127304878 ) ) ;
#2384=AXIS2_PLACEMENT_3D ( 'NONE', #2478, #21008, #4241 ) ;
#2388=CARTESIAN_POINT ( 'NONE',  ( 74.62708615766334219, 133.0342049366344384, -8.851289726714327344 ) ) ;
#2389=CARTESIAN_POINT ( 'NONE',  ( 20.99626426110969390, 137.5292218135913913, 9.918250401459649979 ) ) ;
#2390=FACE_OUTER_BOUND ( 'NONE', #12530, .T. ) ;
#2398=CARTESIAN_POINT ( 'NONE',  ( 9.127117681521182746, 124.1904119534442401, -3.775300622140596030 ) ) ;
#2401=CARTESIAN_POINT ( 'NONE',  ( 9.231363607564425422, 125.4582397780895633, 16.26765482522027639 ) ) ;
#2403=CARTESIAN_POINT ( 'NONE',  ( 0.000000000000000000, 0.000000000000000000, 0.000000000000000000 ) ) ;
#2407=CARTESIAN_POINT ( 'NONE',  ( 77.31131846045057898, 118.9338434746808844, -2.379532457331845485 ) ) ;
#2412=CARTESIAN_POINT ( 'NONE',  ( 14.73996261871784341, 120.6514404024884755, 15.19984638209844441 ) ) ;
#2422=CARTESIAN_POINT ( 'NONE',  ( 70.19721620597543676, 127.0927327670264475, -7.624900598222268400 ) ) ;
#2435=CARTESIAN_POINT ( 'NONE',  ( 29.59780345622613851, 88.32329120701308511, 6.787350155335245994 ) ) ;
#2441=CARTESIAN_POINT ( 'NONE',  ( 70.84063976188440392, 115.3547488198113200, -1.153064885589385025 ) ) ;
#2449=CARTESIAN_POINT ( 'NONE',  ( 45.29500579500201951, 154.0643053174194961, 10.91066218119221709 ) ) ;
#2459=CARTESIAN_POINT ( 'NONE',  ( 44.41273964558330789, 85.70220254879866673, -6.708519844216274564 ) ) ;
#2465=CARTESIAN_POINT ( 'NONE',  ( 57.55288598684787615, 89.00415807515548750, -6.156345639627279986 ) ) ;
#2467=DIRECTION ( 'NONE',  ( 0.000000000000000000, 0.000000000000000000, -1.000000000000000000 ) ) ;
#2478=CARTESIAN_POINT ( 'NONE',  ( 43.01140435219951996, 119.9070776186055838, -35.00000000000000000 ) ) ;
#2484=CARTESIAN_POINT ( 'NONE',  ( 71.26135857449716582, 118.5824631887579272, 4.723566274445706092 ) ) ;
#2491=CARTESIAN_POINT ( 'NONE',  ( 73.32203938827501588, 103.9946350594383517, -0.8753108214479579097 ) ) ;
#2492=CARTESIAN_POINT ( 'NONE',  ( 69.68673170630326297, 129.0522134326295145, 12.29911014595921692 ) ) ;
#2502=CARTESIAN_POINT ( 'NONE',  ( 76.87285023715404009, 124.3600315475450486, -0.5611826874715375446 ) ) ;
#2504=CARTESIAN_POINT ( 'NONE',  ( 12.43312601512511151, 135.2277911470865490, 16.60371454366222466 ) ) ;
#2510=CARTESIAN_POINT ( 'NONE',  ( 9.433072040199128594, 112.8364229897773470, 7.858512901693939234 ) ) ;
#2516=CARTESIAN_POINT ( 'NONE',  ( 21.79768317403592803, 101.2052074350461339, 14.36631359211887649 ) ) ;
#2530=CARTESIAN_POINT ( 'NONE',  ( 20.44379504597808861, 136.6827000062168338, -10.12478428749056469 ) ) ;
#2532=CARTESIAN_POINT ( 'NONE',  ( 44.63189717924443300, 144.8563245053103401, 38.95199156105033467 ) ) ;
#2537=CARTESIAN_POINT ( 'NONE',  ( 44.41273964558330789, 85.70220254879866673, -6.708519844216274564 ) ) ;
#2543=CARTESIAN_POINT ( 'NONE',  ( 47.27474595639033339, 153.9548969447091906, 2.977729283044022957 ) ) ;
#2550=CARTESIAN_POINT ( 'NONE',  ( 58.43892221570314405, 143.5117748958429047, 4.561220828673259398 ) ) ;
#2557=CARTESIAN_POINT ( 'NONE',  ( 68.29446192123552350, 96.82662215664792882, 13.41040346623746515 ) ) ;
#2558=CARTESIAN_POINT ( 'NONE',  ( 38.67087568172628664, 95.28607559046729136, 36.71405245301004783 ) ) ;
#2567=CARTESIAN_POINT ( 'NONE',  ( 23.23160898551418185, 147.7622765488190453, -10.85157364460736140 ) ) ;
#2588=CARTESIAN_POINT ( 'NONE',  ( 29.27693512915957541, 95.18479568265063051, 6.985315079919499404 ) ) ;
#2594=CARTESIAN_POINT ( 'NONE',  ( 11.67247064774405452, 106.1322524520788875, 1.624861436118421043 ) ) ;
#2595=CARTESIAN_POINT ( 'NONE',  ( 32.21091799184858218, 93.94358800413606048, -12.14875741943239085 ) ) ;
#2596=CARTESIAN_POINT ( 'NONE',  ( 10.42839491720816625, 130.4056617841633283, -4.565575592310756825 ) ) ;
#2607=CARTESIAN_POINT ( 'NONE',  ( 27.13677837140323490, 150.1474281128565167, -2.704124018797368301 ) ) ;
#2614=CARTESIAN_POINT ( 'NONE',  ( 13.37233465371036090, 102.6159639102351093, 7.501340520787425525 ) ) ;
#2620=CARTESIAN_POINT ( 'NONE',  ( 64.30534519084480394, 138.3942263399134447, -9.129458798097310535 ) ) ;
#2621=( NAMED_UNIT ( * ) PLANE_ANGLE_UNIT ( ) SI_UNIT ( $, .RADIAN. ) );
#2631=CARTESIAN_POINT ( 'NONE',  ( 65.16383128666855384, 137.2272505635282585, -1.077070130972596962 ) ) ;
#2633=CARTESIAN_POINT ( 'NONE',  ( 48.01156915178761864, 144.4019414068667686, 34.53828804502998651 ) ) ;
#2646=CARTESIAN_POINT ( 'NONE',  ( 32.75162935850930523, 152.6515011162663313, 2.501635869428501469 ) ) ;
#2652=CARTESIAN_POINT ( 'NONE',  ( 58.92189266798492042, 143.1894642327317513, 11.58510527907202992 ) ) ;
#2653=ORIENTED_EDGE ( 'NONE', *, *, #14566, .F. ) ;
#2659=CARTESIAN_POINT ( 'NONE',  ( 69.83118287335672392, 141.1824132108841638, 4.838974892866481525 ) ) ;
#2660=CARTESIAN_POINT ( 'NONE',  ( 41.70806931348493407, 94.93898644073527748, 39.04902473919937478 ) ) ;
#2670=CARTESIAN_POINT ( 'NONE',  ( 74.62708615766334219, 133.0342049366344384, -8.851289726714327344 ) ) ;
#2680=VERTEX_POINT ( 'NONE', #15549 ) ;
#2689=STYLED_ITEM ( 'NONE', ( #6670 ), #14549 ) ;
#2698=CARTESIAN_POINT ( 'NONE',  ( 62.38482844916680392, 99.30468409114129713, 12.58043553469319953 ) ) ;
#2701=CARTESIAN_POINT ( 'NONE',  ( 43.01140435219951996, 119.9070776186055838, -35.00000000000000000 ) ) ;
#2705=CARTESIAN_POINT ( 'NONE',  ( 25.52397925108762067, 90.47728371212039633, 7.934596195134201224 ) ) ;
#2707=CARTESIAN_POINT ( 'NONE',  ( 52.12662541604375122, 146.5080492276505311, -15.72009227599853531 ) ) ;
#2709=CARTESIAN_POINT ( 'NONE',  ( 32.98198692859195802, 152.6383102900375093, -3.493975233523312962 ) ) ;
#2712=ORIENTED_EDGE ( 'NONE', *, *, #19599, .F. ) ;
#2718=CARTESIAN_POINT ( 'NONE',  ( 17.52322149637394233, 97.17389352242535949, -4.727774211004094340 ) ) ;
#2722=CARTESIAN_POINT ( 'NONE',  ( 24.41145734808947054, 148.6458414325078081, 10.19629000755267434 ) ) ;
#2729=CARTESIAN_POINT ( 'NONE',  ( 66.97354912532109950, 95.34500505098478129, 5.477698430975745048 ) ) ;
#2735=CARTESIAN_POINT ( 'NONE',  ( 32.03768905382736421, 145.5187656067679711, 23.43402463578956585 ) ) ;
#2747=CARTESIAN_POINT ( 'NONE',  ( 26.96882349746146446, 96.81297435472995971, -11.91061488385382106 ) ) ;
#2755=CARTESIAN_POINT ( 'NONE',  ( 20.91437931538276374, 145.9617080342048894, -10.94665030085253044 ) ) ;
#2763=CARTESIAN_POINT ( 'NONE',  ( 59.95958160670890180, 90.07020311440788873, 19.76341270931769500 ) ) ;
#2778=CARTESIAN_POINT ( 'NONE',  ( 52.46025766099742071, 152.8098426157893925, 11.14871012209260748 ) ) ;
#2785=CARTESIAN_POINT ( 'NONE',  ( 10.91571581598819662, 131.8149664739095783, 9.482090752819161139 ) ) ;
#2811=CARTESIAN_POINT ( 'NONE',  ( 35.68099593698222094, 147.2217917141817907, 16.62841781073025871 ) ) ;
#2817=CARTESIAN_POINT ( 'NONE',  ( 8.927628897234525240, 116.7075971571176751, 1.981832035706394546 ) ) ;
#2818=CARTESIAN_POINT ( 'NONE',  ( 26.92635752117756098, 142.9018661569831750, -16.76761354414967542 ) ) ;
#2825=CARTESIAN_POINT ( 'NONE',  ( 23.23160898551418185, 147.7622765488190453, -10.85157364460736140 ) ) ;
#2830=( NAMED_UNIT ( * ) PLANE_ANGLE_UNIT ( ) SI_UNIT ( $, .RADIAN. ) );
#2834=CARTESIAN_POINT ( 'NONE',  ( 55.35048440753327981, 87.88826800209452017, -1.070088050731120344 ) ) ;
#2840=CARTESIAN_POINT ( 'NONE',  ( 71.17671054099098171, 117.3556635612232810, 18.77100214853170357 ) ) ;
#2849=CARTESIAN_POINT ( 'NONE',  ( 56.57648482392179545, 95.27494636639178793, 7.851242587554376762 ) ) ;
#2859=CARTESIAN_POINT ( 'NONE',  ( 69.71972837475884432, 98.49221204361529658, -7.660766391518695428 ) ) ;
#2867=CARTESIAN_POINT ( 'NONE',  ( 74.43934690056714487, 106.1333445020626129, 19.04903893889577660 ) ) ;
#2871=CARTESIAN_POINT ( 'NONE',  ( 77.09984031027478579, 117.8059907461747429, -7.347010041119995449 ) ) ;
#2883=CARTESIAN_POINT ( 'NONE',  ( 27.67177345608778793, 143.5689829720894011, 10.27550654291302479 ) ) ;
#2886=CARTESIAN_POINT ( 'NONE',  ( 51.78234217841457365, 152.9971814535558963, 4.124977536042813142 ) ) ;
#2899=CARTESIAN_POINT ( 'NONE',  ( 10.16827731527805767, 110.2528774685086574, 8.767718578943870966 ) ) ;
#2923=CARTESIAN_POINT ( 'NONE',  ( 29.27949416537561333, 144.5119445999418986, 23.32977622066093204 ) ) ;
#2928=CYLINDRICAL_SURFACE ( 'NONE', #11527, 4.999999999999997335 ) ;
#2929=CARTESIAN_POINT ( 'NONE',  ( 72.98789752971651978, 103.3738663174133023, 6.148623012889737005 ) ) ;
#2930=CARTESIAN_POINT ( 'NONE',  ( 69.30627838890079317, 109.9422389716749535, -13.93421298911417416 ) ) ;
#2943=CARTESIAN_POINT ( 'NONE',  ( 13.97286934428321103, 138.1879231288898495, 15.71574578848041881 ) ) ;
#2950=CARTESIAN_POINT ( 'NONE',  ( 15.78326802858598299, 112.2624592280589439, 21.86641499745291028 ) ) ;
#2961=CARTESIAN_POINT ( 'NONE',  ( 42.16380956469475194, 91.80013758078052888, 8.446644326836734606 ) ) ;
#2964=DIRECTION ( 'NONE',  ( -1.000000000000000000, 0.000000000000000000, 0.000000000000000000 ) ) ;
#2971=CARTESIAN_POINT ( 'NONE',  ( 75.80354157443048280, 110.0810758630161672, 5.910575721798123183 ) ) ;
#2979=CARTESIAN_POINT ( 'NONE',  ( 8.737656864016759783, 121.5850998216562431, 22.14420391595633220 ) ) ;
#2983=CARTESIAN_POINT ( 'NONE',  ( 69.52170837389681424, 98.37355370181180092, -13.65637406972050272 ) ) ;
#2986=CARTESIAN_POINT ( 'NONE',  ( 69.85845278386915425, 111.2786852186620621, 13.01367670771671747 ) ) ;
#2991=CARTESIAN_POINT ( 'NONE',  ( 31.84750084766683287, 94.01163676417708359, 0.8705387173494113506 ) ) ;
#2996=CARTESIAN_POINT ( 'NONE',  ( 39.24730198293589467, 95.19097405389743471, 30.90345582088290044 ) ) ;
#3007=CARTESIAN_POINT ( 'NONE',  ( 48.17517050666977241, 153.7480039124125994, 4.005852979123367241 ) ) ;
#3023=DIRECTION ( 'NONE',  ( 0.9387810623359078566, 0.3426822732243069436, 0.03548206049944095664 ) ) ;
#3031=CARTESIAN_POINT ( 'NONE',  ( 32.03768905382736421, 145.5187656067679711, 23.43402463578956585 ) ) ;
#3037=CARTESIAN_POINT ( 'NONE',  ( 15.97061701817242785, 140.8453463817331794, 16.82122940411608170 ) ) ;
#3038=CARTESIAN_POINT ( 'NONE',  ( 14.89151287784495281, 119.8505320279099209, -10.83935810001172229 ) ) ;
#3055=CARTESIAN_POINT ( 'NONE',  ( 52.27439898384277939, 152.9467924839493946, 17.14431721725165758 ) ) ;
#3062=CARTESIAN_POINT ( 'NONE',  ( 31.34884810169724645, 145.5825485123889109, -10.55804779818428862 ) ) ;
#3073=CARTESIAN_POINT ( 'NONE',  ( 65.57965399412842089, 103.1314161556117028, 7.375186511277089352 ) ) ;
#3085=CARTESIAN_POINT ( 'NONE',  ( 66.76198117565915879, 95.25264312590786631, -0.5179092472497510702 ) ) ;
#3093=CARTESIAN_POINT ( 'NONE',  ( 42.43310160994198554, 85.59785666124599857, 20.35848333119881914 ) ) ;
#3097=CARTESIAN_POINT ( 'NONE',  ( 27.13677837140323490, 150.1474281128565167, -2.704124018797368301 ) ) ;
#3100=CARTESIAN_POINT ( 'NONE',  ( 65.77248029998415291, 103.2585056976580091, 13.37079068582577435 ) ) ;
#3106=CARTESIAN_POINT ( 'NONE',  ( 51.84853669763433004, 93.12814091139611605, 7.061107544354192633 ) ) ;
#3108=CARTESIAN_POINT ( 'NONE',  ( 14.48810111090402941, 100.9784058478479523, 15.43442115621699529 ) ) ;
#3115=EDGE_LOOP ( 'NONE', ( #387, #5902 ) ) ;
#3118=CARTESIAN_POINT ( 'NONE',  ( 71.03835150376274044, 100.2492380157770526, 6.267546321443639989 ) ) ;
#3125=CARTESIAN_POINT ( 'NONE',  ( 75.10802748102119608, 108.0013139708956800, -8.018167963582932600 ) ) ;
#3143=CARTESIAN_POINT ( 'NONE',  ( 51.52566954327383542, 92.93877768781105431, 20.08059929855049219 ) ) ;
#3149=CARTESIAN_POINT ( 'NONE',  ( 52.46025766099742071, 152.8098426157893925, 11.14871012209260748 ) ) ;
#3150=CARTESIAN_POINT ( 'NONE',  ( 70.62278752756289180, 114.5844828164671441, -0.1247842873985126749 ) ) ;
#3170=CARTESIAN_POINT ( 'NONE',  ( 77.17837728419731036, 116.7372127726149245, 18.69201499742705153 ) ) ;
#3175=CARTESIAN_POINT ( 'NONE',  ( 70.43474449472395804, 99.54920534645194152, 7.295875980836476593 ) ) ;
#3176=CARTESIAN_POINT ( 'NONE',  ( 69.25106277675128297, 109.5764507715396832, -0.9149236002526208722 ) ) ;
#3187=CARTESIAN_POINT ( 'NONE',  ( 27.89715912807487186, 143.6191053679247602, 4.279900468622926724 ) ) ;
#3198=CARTESIAN_POINT ( 'NONE',  ( 71.03835150376274044, 100.2492380157770526, 6.267546321443639989 ) ) ;
#3205=CARTESIAN_POINT ( 'NONE',  ( 10.15219960346482431, 110.0225462658725490, 14.76332465322822074 ) ) ;
#3208=CARTESIAN_POINT ( 'NONE',  ( 29.26409511065843105, 88.64202804534433255, -5.203872050689020590 ) ) ;
#3216=CARTESIAN_POINT ( 'NONE',  ( 66.10898071834657230, 103.7292514542787245, 6.347102411281516865 ) ) ;
#3228=CARTESIAN_POINT ( 'NONE',  ( 50.92548328124963319, 86.60151408976496157, 0.07716523989554470442 ) ) ;
#3236=CARTESIAN_POINT ( 'NONE',  ( 73.40451243997107156, 135.6611253642151098, -1.946480675884423084 ) ) ;
#3239=CARTESIAN_POINT ( 'NONE',  ( 16.16443657470430750, 128.5343009702184816, -4.486436360144259616 ) ) ;
#3244=CARTESIAN_POINT ( 'NONE',  ( 53.88337135589062399, 152.3674195137575964, -9.803719146365084569 ) ) ;
#3254=CIRCLE ( 'NONE', #21207, 3.000000000000000444 ) ;
#3256=CARTESIAN_POINT ( 'NONE',  ( 18.01452421378985136, 106.6802099491036273, 21.62814552769798837 ) ) ;
#3261=FACE_OUTER_BOUND ( 'NONE', #9156, .T. ) ;
#3262=CARTESIAN_POINT ( 'NONE',  ( 22.01597290215339697, 101.2010103422484519, -4.648787059867797389 ) ) ;
#3279=CARTESIAN_POINT ( 'NONE',  ( 73.69864372527810303, 135.2613471474284097, 11.07306444099484466 ) ) ;
#3284=CARTESIAN_POINT ( 'NONE',  ( 61.89860894053757789, 148.3622700476249463, -1.513601781051955530 ) ) ;
#3286=CARTESIAN_POINT ( 'NONE',  ( 50.21395344324809429, 147.1711500555979626, 4.203964687196366512 ) ) ;
#3298=CARTESIAN_POINT ( 'NONE',  ( 21.19424684193554143, 137.6478987072957807, 3.922641511544080917 ) ) ;
#3309=CARTESIAN_POINT ( 'NONE',  ( 17.14282613681034917, 97.48634091255654255, 8.291567264837656381 ) ) ;
#3317=CARTESIAN_POINT ( 'NONE',  ( 52.31916092102454741, 146.6125112339981627, 3.294994845742023948 ) ) ;
#3327=CARTESIAN_POINT ( 'NONE',  ( 68.29827362630597065, 132.3882971431532383, 5.156253003121209488 ) ) ;
#3335=CARTESIAN_POINT ( 'NONE',  ( 38.51811260612901577, 144.5002972345523631, 36.42795439419948877 ) ) ;
#3340=CARTESIAN_POINT ( 'NONE',  ( 28.65042173108665935, 151.0721679115347911, -4.641026357035400451 ) ) ;
#3346=CARTESIAN_POINT ( 'NONE',  ( 50.33192209904863290, 153.3481575868430014, -9.922832680162505525 ) ) ;
#3349=CARTESIAN_POINT ( 'NONE',  ( 34.72595348466361287, 146.8618156516888291, -3.415175568290148345 ) ) ;
#3356=CARTESIAN_POINT ( 'NONE',  ( 76.20123706073158587, 111.5182621349952257, -8.137091297256032973 ) ) ;
#3367=CARTESIAN_POINT ( 'NONE',  ( 57.86150831142030171, 95.93494642397840266, -0.2007220744356660869 ) ) ;
#3373=FACE_BOUND ( 'NONE', #21625, .T. ) ;
#3374=CARTESIAN_POINT ( 'NONE',  ( 74.27779736592162863, 105.9683817680885056, 13.05343286460986363 ) ) ;
#3375=CARTESIAN_POINT ( 'NONE',  ( 15.79683473163509966, 126.9851207307152521, 3.446356185820485418 ) ) ;
#3393=CARTESIAN_POINT ( 'NONE',  ( 67.29571637068438861, 144.1510613573267108, 10.71565575886252297 ) ) ;
#3398=CARTESIAN_POINT ( 'NONE',  ( 70.84804472268019992, 100.1183116193850964, 0.2719452077637916076 ) ) ;
#3399=CARTESIAN_POINT ( 'NONE',  ( 18.57470074671828542, 105.8336742703428257, 1.585105279193314010 ) ) ;
#3411=CARTESIAN_POINT ( 'NONE',  ( 43.01140435219951996, 119.9070776186055838, 50.00000000000002842 ) ) ;
#3414=CARTESIAN_POINT ( 'NONE',  ( 27.04509496028088478, 143.0549882411833380, 11.23409068567602098 ) ) ;
#3426=CARTESIAN_POINT ( 'NONE',  ( 35.69068542950036260, 86.46542255174357194, 7.577194441455407770 ) ) ;
#3433=CARTESIAN_POINT ( 'NONE',  ( 70.48772827241290884, 113.2068808858050630, -2.062176545857650201 ) ) ;
#3443=CARTESIAN_POINT ( 'NONE',  ( 69.85845278386915425, 111.2786852186620621, 13.01367670771671747 ) ) ;
#3457=CARTESIAN_POINT ( 'NONE',  ( 12.61881386508366809, 104.1535352963828984, 15.55354899318430739 ) ) ;
#3461=DIRECTION ( 'NONE',  ( 1.000000000000000000, 0.000000000000000000, 0.000000000000000000 ) ) ;
#3463=CARTESIAN_POINT ( 'NONE',  ( 69.83118287335672392, 141.1824132108841638, 4.838974892866481525 ) ) ;
#3471=CARTESIAN_POINT ( 'NONE',  ( 59.50342836137831171, 89.99885106877826502, 7.772197353298202493 ) ) ;
#3481=CARTESIAN_POINT ( 'NONE',  ( 32.38101408406643600, 93.78751416920769657, -6.153149741203968404 ) ) ;
#3487=CARTESIAN_POINT ( 'NONE',  ( 77.07719282571002850, 116.5297446719512209, 12.69640610750513865 ) ) ;
#3490=CARTESIAN_POINT ( 'NONE',  ( 17.65293208513390866, 132.0582047407114885, -3.339186312533837242 ) ) ;
#3491=EDGE_CURVE ( 'NONE', #1853, #4221, #21002, .T. ) ;
#3505=CARTESIAN_POINT ( 'NONE',  ( 9.955767346236717330, 110.6995739201198887, 21.78706596723887756 ) ) ;
#3509=CARTESIAN_POINT ( 'NONE',  ( 41.12929731208597417, 154.0090796829547912, -2.227802639778228233 ) ) ;
#3510=CARTESIAN_POINT ( 'NONE',  ( 70.21798013780751546, 127.3226622636268672, -1.629293503064584536 ) ) ;
#3520=CARTESIAN_POINT ( 'NONE',  ( 15.69291839309778958, 99.40984958608130739, -11.63272432674803802 ) ) ;
#3530=CARTESIAN_POINT ( 'NONE',  ( 18.14018356548558941, 143.3940520581896862, 16.92415443696469879 ) ) ;
#3536=CARTESIAN_POINT ( 'NONE',  ( 62.56935518920172967, 140.3353681171158200, 3.771274953561639887 ) ) ;
#3547=CARTESIAN_POINT ( 'NONE',  ( 71.06985403747866314, 121.7623127629220932, -14.41049859375789666 ) ) ;
#3550=LINE ( 'NONE', #6760, #19506 ) ;
#3554=CARTESIAN_POINT ( 'NONE',  ( 38.04343743846316528, 144.4085798130015803, 34.86469163422182049 ) ) ;
#3560=CARTESIAN_POINT ( 'NONE',  ( 28.07864021081662287, 89.10199518432737875, 14.83897397183228861 ) ) ;
#3568=CARTESIAN_POINT ( 'NONE',  ( 63.41425016244589585, 92.41789933959738335, 6.624947895572852019 ) ) ;
#3575=CARTESIAN_POINT ( 'NONE',  ( 20.88913110926514705, 146.0313881486468119, 3.053432864643822686 ) ) ;
#3584=CARTESIAN_POINT ( 'NONE',  ( 16.33471683235446292, 110.7640000046674089, -5.200637885961103102 ) ) ;
#3593=CARTESIAN_POINT ( 'NONE',  ( 65.16383128666855384, 137.2272505635282585, -1.077070130972596962 ) ) ;
#3614=CARTESIAN_POINT ( 'NONE',  ( 51.76721073900363734, 146.7980033588722506, -3.728880589165500137 ) ) ;
#3618=CARTESIAN_POINT ( 'NONE',  ( 51.60797029699607918, 86.77139250312444574, -6.946567135388369785 ) ) ;
#3619=CARTESIAN_POINT ( 'NONE',  ( 43.64334309031418968, 148.0990856179656419, -3.057864931601543823 ) ) ;
#3628=CARTESIAN_POINT ( 'NONE',  ( 47.68298272704948459, 153.7393326413893817, -9.013488496775837078 ) ) ;
#3638=CARTESIAN_POINT ( 'NONE',  ( 34.41316853928974950, 153.0433231119815503, 10.55326060710041958 ) ) ;
#3642=CARTESIAN_POINT ( 'NONE',  ( 69.03752116822961682, 130.9715778530742227, -2.776543650264200025 ) ) ;
#3649=VERTEX_POINT ( 'NONE', #14626 ) ;
#3654=CARTESIAN_POINT ( 'NONE',  ( 25.00529828370466490, 141.4305569644042464, -16.86339438981633876 ) ) ;
#3656=DIRECTION ( 'NONE',  ( 0.000000000000000000, 0.000000000000000000, -1.000000000000000000 ) ) ;
#3665=CARTESIAN_POINT ( 'NONE',  ( 75.40436159597490473, 130.9804297329818326, 12.22031048084446248 ) ) ;
#3671=CARTESIAN_POINT ( 'NONE',  ( 40.90832812944997698, 154.0758954209757121, 3.767805038447253452 ) ) ;
#3681=CARTESIAN_POINT ( 'NONE',  ( 61.01612483116806374, 90.79174121657607088, -0.2798613066081144796 ) ) ;
#3689=CARTESIAN_POINT ( 'NONE',  ( 24.69269415895541542, 98.46806607146707790, -5.796035312751787849 ) ) ;
#3698=CARTESIAN_POINT ( 'NONE',  ( 22.73392375623628681, 139.3438357627746882, 11.01889030017397531 ) ) ;
#3705=B_SPLINE_CURVE_WITH_KNOTS ( 'NONE', 3,
 ( #5406, #3764, #553, #10492, #15548, #17191, #2103, #8841, #7183, #12239, #2313, #3872, #17300, #14535, #14320, #19500, #1204, #17947, #7618, #2633, #21276, #19610, #6154, #9268, #21164, #12889, #990, #20949, #11124, #19393, #21062, #776, #4290, #2532, #4504, #1098, #9489, #11017 ),
 .UNSPECIFIED., .F., .F.,
 ( 4, 2, 2, 2, 2, 2, 2, 2, 2, 2, 2, 2, 2, 2, 2, 2, 2, 2, 4 ),
 ( 0.01567185795944686655, 0.01665109603395608165, 0.01763033410846529675, 0.01811995314571990950, 0.01860957218297452573, 0.01958881025748375124, 0.02056804833199297675, 0.02154728640650219532, 0.02252652448101141389, 0.02350576255552062899, 0.02448500063002984756, 0.02546423870453906613, 0.02644347677904828470, 0.02693309581630289051, 0.02742271485355749633, 0.02840195292806670796, 0.02938119100257591959, 0.03036042907708513122, 0.03133966715159434285 ),
 .UNSPECIFIED. ) ;
#3717=CARTESIAN_POINT ( 'NONE',  ( 17.08493018425929932, 131.2036312357472241, 1.628145005703640624 ) ) ;
#3721=CARTESIAN_POINT ( 'NONE',  ( 23.23160898551418185, 147.7622765488190453, -10.85157364460736140 ) ) ;
#3723=CARTESIAN_POINT ( 'NONE',  ( 50.77370750611731154, 147.0167679772302165, 11.22784935402935957 ) ) ;
#3733=CARTESIAN_POINT ( 'NONE',  ( 13.64837572802379562, 102.4646860582014796, -11.51360178106338594 ) ) ;
#3744=CARTESIAN_POINT ( 'NONE',  ( 74.27779736592162863, 105.9683817680885056, 13.05343286460986363 ) ) ;
#3750=CARTESIAN_POINT ( 'NONE',  ( 53.23527110998836775, 93.53878102080766155, -0.9907194398206048414 ) ) ;
#3762=CARTESIAN_POINT ( 'NONE',  ( 35.06472793454997117, 92.93335285089702325, -12.26792952838020767 ) ) ;
#3764=CARTESIAN_POINT ( 'NONE',  ( 43.33809753620296590, 144.9070776186055696, 29.21067981925357060 ) ) ;
#3767=CARTESIAN_POINT ( 'NONE',  ( 46.77903254544086309, 95.19149378333804634, 30.90720150815159784 ) ) ;
#3775=CARTESIAN_POINT ( 'NONE',  ( 9.976645104453018220, 110.9295780357170571, 15.79146183154218619 ) ) ;
#3780=CARTESIAN_POINT ( 'NONE',  ( 58.57487293839693621, 150.3975950434478648, 4.362879525569486994 ) ) ;
#3782=CARTESIAN_POINT ( 'NONE',  ( 28.62772086389876947, 95.65184626908498444, 8.013395860235284829 ) ) ;
#3791=CARTESIAN_POINT ( 'NONE',  ( 64.11693453485118255, 146.8606268255622638, -2.422805558527139080 ) ) ;
#3808=CARTESIAN_POINT ( 'NONE',  ( 56.57648482392179545, 95.27494636639178793, 7.851242587554376762 ) ) ;
#3825=CARTESIAN_POINT ( 'NONE',  ( 27.23529593042425390, 96.43589704216468306, 0.08059930645588880838 ) ) ;
#3830=CARTESIAN_POINT ( 'NONE',  ( 10.42839491720816625, 130.4056617841633283, -4.565575592310756825 ) ) ;
#3831=CARTESIAN_POINT ( 'NONE',  ( 33.52710748945926866, 93.34978808121778115, 14.79936193957723312 ) ) ;
#3841=CARTESIAN_POINT ( 'NONE',  ( 77.13564277734779751, 118.5067815986552375, -14.37074460762677397 ) ) ;
#3851=CARTESIAN_POINT ( 'NONE',  ( 30.18028515090226449, 151.2280014487717779, 17.43780275515692679 ) ) ;
#3858=CARTESIAN_POINT ( 'NONE',  ( 68.27453032555700929, 132.6178071945132046, 11.15186410612756696 ) ) ;
#3870=CARTESIAN_POINT ( 'NONE',  ( 19.52755003174225124, 104.2962547294809070, 15.51356631106660089 ) ) ;
#3872=CARTESIAN_POINT ( 'NONE',  ( 46.77550672146314525, 144.6231811833137044, 30.90345582088290044 ) ) ;
#3875=CARTESIAN_POINT ( 'NONE',  ( 47.85069476305888259, 95.37983616430958023, 35.51056251760059013 ) ) ;
#3882=CARTESIAN_POINT ( 'NONE',  ( 76.06694498870253085, 129.1134374410657983, 4.287174360044270216 ) ) ;
#3889=CARTESIAN_POINT ( 'NONE',  ( 72.98789752971651978, 103.3738663174133023, 6.148623012889737005 ) ) ;
#3891=CARTESIAN_POINT ( 'NONE',  ( 70.94289844336020678, 123.7826807253454575, 5.513563639855703080 ) ) ;
#3898=CARTESIAN_POINT ( 'NONE',  ( 64.59149290518072917, 93.33317027722591774, -7.422718449586769296 ) ) ;
#3915=CARTESIAN_POINT ( 'NONE',  ( 15.29689364450883815, 124.6620785063593786, 10.35143954082134954 ) ) ;
#3930=CARTESIAN_POINT ( 'NONE',  ( 22.02512380705847406, 92.75866610308527527, 21.07306443996510481 ) ) ;
#3936=CARTESIAN_POINT ( 'NONE',  ( 28.88048086162541850, 151.0887240815949895, -10.63664014359656385 ) ) ;
#3937=CARTESIAN_POINT ( 'NONE',  ( 19.23080508249268661, 135.0620028898917440, 9.799277925644819476 ) ) ;
#3949=CARTESIAN_POINT ( 'NONE',  ( 8.933461960486459574, 117.6319094064757422, 3.010161695468211551 ) ) ;
#3951=CARTESIAN_POINT ( 'NONE',  ( 18.14018356548558941, 143.3940520581896862, 16.92415443696469879 ) ) ;
#3961=CARTESIAN_POINT ( 'NONE',  ( 24.41145734808947054, 148.6458414325078081, 10.19629000755267434 ) ) ;
#3967=CARTESIAN_POINT ( 'NONE',  ( 22.35924357203464297, 139.2281224154095014, 9.009280560090923373 ) ) ;
#3977=CARTESIAN_POINT ( 'NONE',  ( 62.76710561173204894, 139.9178416638646638, -8.219927273936241008 ) ) ;
#3984=CARTESIAN_POINT ( 'NONE',  ( 47.49650721231805761, 95.31256562107512309, 31.99467674420385777 ) ) ;
#3991=CARTESIAN_POINT ( 'NONE',  ( 10.61292492956169475, 108.6005711365770026, 0.7156557588857267449 ) ) ;
#3998=CARTESIAN_POINT ( 'NONE',  ( 62.17156016504299032, 99.21662021101468554, 6.584824431686855384 ) ) ;
#4003=CARTESIAN_POINT ( 'NONE',  ( 66.76198117565915879, 95.25264312590786631, -0.5179092472497510702 ) ) ;
#4013=CARTESIAN_POINT ( 'NONE',  ( 28.88048086162541850, 151.0887240815949895, -10.63664014359656385 ) ) ;
#4019=CARTESIAN_POINT ( 'NONE',  ( 15.82502354501850483, 112.7224674592991818, 9.875206726065272278 ) ) ;
#4038=CARTESIAN_POINT ( 'NONE',  ( 37.44377528459369131, 147.6348322250013894, 2.699600794211013621 ) ) ;
#4042=ORIENTED_EDGE ( 'NONE', *, *, #17003, .T. ) ;
#4044=CARTESIAN_POINT ( 'NONE',  ( 77.15313604554262383, 122.4041478163663612, -8.494263314424808087 ) ) ;
#4045=CARTESIAN_POINT ( 'NONE',  ( 68.29827362630597065, 132.3882971431532383, 5.156253003121209488 ) ) ;
#4054=CARTESIAN_POINT ( 'NONE',  ( 25.98494354700934750, 90.29984025740714060, -5.084945496952688160 ) ) ;
#4056=CARTESIAN_POINT ( 'NONE',  ( 19.13088699441526686, 95.37848931739559077, 15.19637875606281341 ) ) ;
#4061=CARTESIAN_POINT ( 'NONE',  ( 73.49404125747247463, 104.1488224428393039, 5.120290292223307560 ) ) ;
#4064=PLANE ( 'NONE',  #13238 ) ;
#4069=CARTESIAN_POINT ( 'NONE',  ( 50.02529374262071826, 147.3041493969045064, 10.19957357710909207 ) ) ;
#4080=CARTESIAN_POINT ( 'NONE',  ( 67.81612255856859406, 106.6615363072494915, -6.791355845220972576 ) ) ;
#4093=CARTESIAN_POINT ( 'NONE',  ( 33.74677389505396263, 86.86730044589080535, -0.3555069876874490942 ) ) ;
#4100=CARTESIAN_POINT ( 'NONE',  ( 22.56676867748217674, 139.3294883087844198, 3.013676707730225779 ) ) ;
#4107=CARTESIAN_POINT ( 'NONE',  ( 76.92284642892752800, 124.5854180935290714, 5.434424407683230207 ) ) ;
#4118=CARTESIAN_POINT ( 'NONE',  ( 26.28921445626723852, 149.7786157371718616, -3.732453678475698311 ) ) ;
#4125=CARTESIAN_POINT ( 'NONE',  ( 16.85323768375146614, 130.1535925207217588, 10.57871716905499682 ) ) ;
#4144=CARTESIAN_POINT ( 'NONE',  ( 55.43026649837064213, 94.49908577724413306, 5.913859291446645905 ) ) ;
#4153=CARTESIAN_POINT ( 'NONE',  ( 75.16956835342354282, 131.6452004531123805, 5.196376467030073165 ) ) ;
#4154=CARTESIAN_POINT ( 'NONE',  ( 44.86974823489592978, 148.0457227541334362, 10.98970740178311090 ) ) ;
#4164=CARTESIAN_POINT ( 'NONE',  ( 75.16838608161717161, 131.4143534805274101, -0.7992312111982662337 ) ) ;
#4166=CARTESIAN_POINT ( 'NONE',  ( 38.54497605562327323, 85.96704844161884296, 14.48200433579215662 ) ) ;
#4171=CARTESIAN_POINT ( 'NONE',  ( 66.79148812173782801, 144.6461433805978061, 3.691718863876278345 ) ) ;
#4178=CARTESIAN_POINT ( 'NONE',  ( 69.49514557983670215, 129.8286863358667347, 11.27102936561352742 ) ) ;
#4188=CARTESIAN_POINT ( 'NONE',  ( 70.72621728061167801, 115.1542034346632875, -7.148670959876664455 ) ) ;
#4195=CARTESIAN_POINT ( 'NONE',  ( 51.60797029699607918, 86.77139250312444574, -6.946567135388369785 ) ) ;
#4200=CARTESIAN_POINT ( 'NONE',  ( 57.78537588620154963, 150.8774031240512272, 3.334753224648476788 ) ) ;
#4206=CARTESIAN_POINT ( 'NONE',  ( 29.72792815944318789, 144.7825833525567134, 3.370790685444458479 ) ) ;
#4214=CARTESIAN_POINT ( 'NONE',  ( 48.17517050666977241, 153.7480039124125994, 4.005852979123367241 ) ) ;
#4215=CARTESIAN_POINT ( 'NONE',  ( 38.51754685674856660, 95.31395939335972400, 36.42700876960375922 ) ) ;
#4221=VERTEX_POINT ( 'NONE', #20906 ) ;
#4225=CARTESIAN_POINT ( 'NONE',  ( 39.42188022582085694, 153.9507182763122159, -10.27990332573616961 ) ) ;
#4241=DIRECTION ( 'NONE',  ( -1.000000000000000000, 0.000000000000000000, 0.000000000000000000 ) ) ;
#4247=CARTESIAN_POINT ( 'NONE',  ( 15.40311202476076780, 126.0397005259128065, 8.413886508562818278 ) ) ;
#4253=CARTESIAN_POINT ( 'NONE',  ( 77.22939692449374149, 120.9137088693742044, 5.553548964694690504 ) ) ;
#4254=CARTESIAN_POINT ( 'NONE',  ( 26.83015598135647295, 142.9878415585355071, 17.22988066553158149 ) ) ;
#4264=CARTESIAN_POINT ( 'NONE',  ( 76.77449255912956971, 125.0547954796211485, -7.584917068115353267 ) ) ;
#4266=CARTESIAN_POINT ( 'NONE',  ( 42.21854335081802390, 85.68333463812091111, 14.36287948008016890 ) ) ;
#4271=CARTESIAN_POINT ( 'NONE',  ( 8.843693174888816344, 123.0768258502195067, 1.191984145255910787 ) ) ;
#4276=CARTESIAN_POINT ( 'NONE',  ( 65.02109649036992778, 137.6666368931563227, 10.91413209638136728 ) ) ;
#4288=CARTESIAN_POINT ( 'NONE',  ( 34.95631105476920197, 146.8486248254830855, -9.410786671241964996 ) ) ;
#4290=CARTESIAN_POINT ( 'NONE',  ( 45.23316362766301779, 144.8099831305763985, 38.70176206714168643 ) ) ;
#4295=CARTESIAN_POINT ( 'NONE',  ( 32.31036143884366396, 152.4250368413922274, -10.51794503956956817 ) ) ;
#4302=CARTESIAN_POINT ( 'NONE',  ( 9.585575214713108139, 112.1464265272871188, 0.8345760063739874335 ) ) ;
#4310=CARTESIAN_POINT ( 'NONE',  ( 19.23080508249268661, 135.0620028898917440, 9.799277925644819476 ) ) ;
#4317=CARTESIAN_POINT ( 'NONE',  ( 58.57487293839693621, 150.3975950434478648, 4.362879525569486994 ) ) ;
#4326=CARTESIAN_POINT ( 'NONE',  ( 64.59149290518072917, 93.33317027722591774, -7.422718449586769296 ) ) ;
#4347=CARTESIAN_POINT ( 'NONE',  ( 70.16915148685765757, 112.0176666281686977, 11.98539833154344691 ) ) ;
#4353=CARTESIAN_POINT ( 'NONE',  ( 32.14050509837299785, 87.44534670509604268, 7.696117750009315195 ) ) ;
#4354=CARTESIAN_POINT ( 'NONE',  ( 15.16534570839878349, 115.4582699162533288, 15.98979919289822149 ) ) ;
#4355=CARTESIAN_POINT ( 'NONE',  ( 77.15313604554262383, 122.4041478163663612, -8.494263314424808087 ) ) ;
#4365=CARTESIAN_POINT ( 'NONE',  ( 12.20328755962376199, 134.6477104347696923, -3.418325544530929516 ) ) ;
#4372=CARTESIAN_POINT ( 'NONE',  ( 64.81014823317600815, 93.40725510594978687, -1.427111354441281899 ) ) ;
#4379=CARTESIAN_POINT ( 'NONE',  ( 15.11992972970532279, 115.2318815533876375, 21.98540506394948224 ) ) ;
#4385=ORIENTED_EDGE ( 'NONE', *, *, #10963, .T. ) ;
#4390=CARTESIAN_POINT ( 'NONE',  ( 18.53657114080759527, 106.0614633106838909, -4.410498573173142312 ) ) ;
#4392=FACE_OUTER_BOUND ( 'NONE', #9072, .T. ) ;
#4398=CARTESIAN_POINT ( 'NONE',  ( 64.11693453485118255, 146.8606268255622638, -2.422805558527139080 ) ) ;
#4405=CARTESIAN_POINT ( 'NONE',  ( 13.97286934428321103, 138.1879231288898495, 15.71574578848041881 ) ) ;
#4421=CARTESIAN_POINT ( 'NONE',  ( 75.80354157443048280, 110.0810758630161672, 5.910575721798123183 ) ) ;
#4422=CARTESIAN_POINT ( 'NONE',  ( 43.01140435219951286, 94.90707761860558378, 39.21067981925356349 ) ) ;
#4425=CARTESIAN_POINT ( 'NONE',  ( 43.01140435219952707, 144.9070776186055696, 39.21067981925356349 ) ) ;
#4429=CARTESIAN_POINT ( 'NONE',  ( 17.14282613681034917, 97.48634091255654255, 8.291567264837656381 ) ) ;
#4441=AXIS2_PLACEMENT_3D ( 'NONE', #15688, #19009, #7766 ) ;
#4454=CARTESIAN_POINT ( 'NONE',  ( 71.27174135432656499, 120.9783100490299574, 11.62814500561148456 ) ) ;
#4460=CARTESIAN_POINT ( 'NONE',  ( 76.04618105687035268, 128.8835079444423286, -1.708432735116285350 ) ) ;
#4462=CARTESIAN_POINT ( 'NONE',  ( 66.54750331441660194, 135.2948500229566093, -7.982215242636039321 ) ) ;
#4472=CARTESIAN_POINT ( 'NONE',  ( 26.87026879109711786, 150.0197496251087728, 11.30891725959585159 ) ) ;
#4481=CARTESIAN_POINT ( 'NONE',  ( 40.94072057685551869, 85.65469043817564909, -0.5939954219232065347 ) ) ;
#4488=ADVANCED_FACE ( 'NONE', ( #12959 ), #2928, .F. ) ;
#4489=CARTESIAN_POINT ( 'NONE',  ( 66.79315400704923888, 104.7533658121278819, -7.700889860664787534 ) ) ;
#4501=CARTESIAN_POINT ( 'NONE',  ( 63.64508858465791974, 100.8029030738736225, 7.494358438614500351 ) ) ;
#4504=CARTESIAN_POINT ( 'NONE',  ( 44.31473939091409875, 144.8751687964759469, 39.04902473919937478 ) ) ;
#4507=EDGE_CURVE ( 'NONE', #3649, #19172, #20029, .T. ) ;
#4511=CARTESIAN_POINT ( 'NONE',  ( 75.85495621331871519, 129.5603373922052697, -8.732165470513974626 ) ) ;
#4520=CARTESIAN_POINT ( 'NONE',  ( 76.43728072391715500, 127.6653364257898744, 18.33484128816649772 ) ) ;
#4523=CARTESIAN_POINT ( 'NONE',  ( 54.72474920843421131, 151.9887481548900325, -8.775581469602226292 ) ) ;
#4534=CARTESIAN_POINT ( 'NONE',  ( 8.798315742295939046, 121.0924013121165075, 9.124689178586496752 ) ) ;
#4535=CARTESIAN_POINT ( 'NONE',  ( 42.35941266477436784, 94.91347937787368494, 29.24238570022250983 ) ) ;
#4544=CARTESIAN_POINT ( 'NONE',  ( 42.92180000979148957, 85.67454126555050209, 7.339147150375312734 ) ) ;
#4569=CARTESIAN_POINT ( 'NONE',  ( 41.61464536962099459, 148.1530905165343768, 16.86614982034995691 ) ) ;
#4575=CARTESIAN_POINT ( 'NONE',  ( 75.80354157443048280, 110.0810758630161672, 5.910575721798123183 ) ) ;
#4576=CARTESIAN_POINT ( 'NONE',  ( 35.06472793454997117, 92.93335285089702325, -12.26792952838020767 ) ) ;
#4593=ADVANCED_FACE ( 'NONE', ( #3373, #3261 ), #10097, .F. ) ;
#4595=CARTESIAN_POINT ( 'NONE',  ( 10.76517401744387215, 131.6399553617083029, 15.47769843104460463 ) ) ;
#4601=CARTESIAN_POINT ( 'NONE',  ( 15.06790588970514833, 124.2609462974868677, 22.34264618625151044 ) ) ;
#4606=ORIENTED_EDGE ( 'NONE', *, *, #333, .F. ) ;
#4611=CARTESIAN_POINT ( 'NONE',  ( 19.79626631456835284, 104.0394230781280669, 2.494070082984220171 ) ) ;
#4622=CARTESIAN_POINT ( 'NONE',  ( 77.22939692449374149, 120.9137088693742044, 5.553548964694690504 ) ) ;
#4630=CARTESIAN_POINT ( 'NONE',  ( 11.40453246296876877, 106.5480838228176452, 14.64419766361223552 ) ) ;
#4633=CARTESIAN_POINT ( 'NONE',  ( 74.70172802024292480, 107.1710682803345662, -6.989838304517381751 ) ) ;
#4639=CARTESIAN_POINT ( 'NONE',  ( 53.64127281404707048, 146.0262708631457542, 11.34682183016344403 ) ) ;
#4646=CARTESIAN_POINT ( 'NONE',  ( 34.07414013685151843, 93.16113583794900421, 7.775673839875955728 ) ) ;
#4649=CARTESIAN_POINT ( 'NONE',  ( 39.70842430446096216, 95.12513732185091442, 30.44285285587857004 ) ) ;
#4661=CARTESIAN_POINT ( 'NONE',  ( 21.43032318156618388, 146.4805633285969861, 10.07716523980869816 ) ) ;
#4682=CARTESIAN_POINT ( 'NONE',  ( 15.94687047784549172, 111.7036002239776451, 14.84254118869207417 ) ) ;
#4687=CARTESIAN_POINT ( 'NONE',  ( 68.29446192123552350, 96.82662215664792882, 13.41040346623746515 ) ) ;
#4688=CARTESIAN_POINT ( 'NONE',  ( 17.40773937504753377, 131.5336607133424991, -10.36307277412196903 ) ) ;
#4704=CARTESIAN_POINT ( 'NONE',  ( 41.39294982251618649, 154.1830292177732531, 16.78735015533800734 ) ) ;
#4711=CARTESIAN_POINT ( 'NONE',  ( 51.52566954327383542, 92.93877768781105431, 20.08059929855049219 ) ) ;
#4720=CARTESIAN_POINT ( 'NONE',  ( 25.97839122281734703, 97.53232036182296838, 2.136956866322798021 ) ) ;
#4724=FACE_BOUND ( 'NONE', #8639, .T. ) ;
#4732=CARTESIAN_POINT ( 'NONE',  ( 29.43094928344231320, 88.48265962617873015, 0.7917390523231137012 ) ) ;
#4738=CARTESIAN_POINT ( 'NONE',  ( 17.22388115030108224, 97.27017246186569821, 14.28717435998666296 ) ) ;
#4741=CARTESIAN_POINT ( 'NONE',  ( 47.07528247981900904, 85.99676402675389397, -5.799316066731655006 ) ) ;
#4744=CARTESIAN_POINT ( 'NONE',  ( 69.68673170630326297, 129.0522134326295145, 12.29911014595921692 ) ) ;
#4750=CARTESIAN_POINT ( 'NONE',  ( 22.56676867748217674, 139.3294883087844198, 3.013676707730225779 ) ) ;
#4763=CARTESIAN_POINT ( 'NONE',  ( 30.90322180743143576, 151.9278386122780375, 10.43433729856376502 ) ) ;
#4771=CARTESIAN_POINT ( 'NONE',  ( 15.39564893635072806, 140.1373336744895255, -4.208549045858890558 ) ) ;
#4791=CARTESIAN_POINT ( 'NONE',  ( 34.17400395940548918, 146.6865494356538875, -10.43883331896520694 ) ) ;
#4798=CARTESIAN_POINT ( 'NONE',  ( 36.80677928932056631, 92.47987693618573246, 1.660900796654692702 ) ) ;
#4816=CARTESIAN_POINT ( 'NONE',  ( 72.28893465744093305, 137.8051215927966382, 17.97743314940082371 ) ) ;
#4821=CARTESIAN_POINT ( 'NONE',  ( 70.33053884415087964, 140.4045759698336724, 5.867304552604015733 ) ) ;
#4823=CARTESIAN_POINT ( 'NONE',  ( 17.24633477965345918, 131.3686459745448758, -4.367463884209165315 ) ) ;
#4826=ORIENTED_EDGE ( 'NONE', *, *, #5300, .F. ) ;
#4834=CARTESIAN_POINT ( 'NONE',  ( 42.74273477336613780, 91.78896094402264794, 1.422757611514577247 ) ) ;
#4846=CARTESIAN_POINT ( 'NONE',  ( 12.03843011909301453, 134.4860913190374561, 2.577281550626734141 ) ) ;
#4848=AXIS2_PLACEMENT_3D ( 'NONE', #8452, #5133, #170 ) ;
#4854=CARTESIAN_POINT ( 'NONE',  ( 25.66908397218059790, 90.29788686741908066, 13.93020729814628744 ) ) ;
#4858=CARTESIAN_POINT ( 'NONE',  ( 11.90670198672629354, 134.0117795012786814, -10.44205992529839122 ) ) ;
#4867=CARTESIAN_POINT ( 'NONE',  ( 37.56771007382699423, 92.23784766911828115, 0.6328166970475824771 ) ) ;
#4875=CARTESIAN_POINT ( 'NONE',  ( 40.50102589165841493, 144.7822066801371932, 29.87433574750618703 ) ) ;
#4880=CARTESIAN_POINT ( 'NONE',  ( 30.24639091383375700, 151.6717570033048048, 3.410403464249057492 ) ) ;
#4886=CARTESIAN_POINT ( 'NONE',  ( 63.55746018358933469, 147.2895578332197033, -9.446739241148069510 ) ) ;
#4888=CARTESIAN_POINT ( 'NONE',  ( 64.30534519084480394, 138.3942263399134447, -9.129458798097310535 ) ) ;
#4896=CARTESIAN_POINT ( 'NONE',  ( 50.33192209904863290, 153.3481575868430014, -9.922832680162505525 ) ) ;
#4908=CARTESIAN_POINT ( 'NONE',  ( 42.59292608294269655, 91.62918162712271908, 20.43785202907404752 ) ) ;
#4915=CARTESIAN_POINT ( 'NONE',  ( 12.43312601512511151, 135.2277911470865490, 16.60371454366222466 ) ) ;
#4917=CARTESIAN_POINT ( 'NONE',  ( 50.40261314387542768, 147.0381507142914188, -1.791644202716362821 ) ) ;
#4936=CARTESIAN_POINT ( 'NONE',  ( 37.02312590732701381, 153.6946607573816834, 9.644493012478044136 ) ) ;
#4941=CARTESIAN_POINT ( 'NONE',  ( 32.47916914626341622, 146.0660553311768979, 3.489959554161691013 ) ) ;
#4953=CARTESIAN_POINT ( 'NONE',  ( 71.13077487245369923, 119.9619191372588034, 6.660813687590150245 ) ) ;
#4964=CARTESIAN_POINT ( 'NONE',  ( 10.16827731527805767, 110.2528774685086574, 8.767718578943870966 ) ) ;
#4970=CARTESIAN_POINT ( 'NONE',  ( 26.46568392313936968, 149.8720644322279725, 23.30118661649528633 ) ) ;
#4973=CARTESIAN_POINT ( 'NONE',  ( 25.98494354700934750, 90.29984025740714060, -5.084945496952688160 ) ) ;
#4983=CARTESIAN_POINT ( 'NONE',  ( 16.97565887011968400, 109.0741130153051444, 8.727962422049884594 ) ) ;
#4986=CARTESIAN_POINT ( 'NONE',  ( 21.90415124324598750, 92.95514585177724598, 15.07745334355238676 ) ) ;
#4990=CARTESIAN_POINT ( 'NONE',  ( 39.03837758695365778, 144.5900556825055219, 37.26405200954400954 ) ) ;
#4991=DIRECTION ( 'NONE',  ( -0.3428981916074304581, 0.9393725726208712601, 0.000000000000000000 ) ) ;
#4995=CARTESIAN_POINT ( 'NONE',  ( 53.70366401737062034, 152.5123965792994625, -3.808113302951443568 ) ) ;
#4997=VERTEX_POINT ( 'NONE', #10847 ) ;
#5005=CARTESIAN_POINT ( 'NONE',  ( 59.92122946415073415, 142.4742691614619332, -9.367183195626855863 ) ) ;
#5011=CARTESIAN_POINT ( 'NONE',  ( 75.85495621331871519, 129.5603373922052697, -8.732165470513974626 ) ) ;
#5022=CARTESIAN_POINT ( 'NONE',  ( 69.25106277675128297, 109.5764507715396832, -0.9149236002526208722 ) ) ;
#5028=CARTESIAN_POINT ( 'NONE',  ( 34.41316853928974950, 153.0433231119815503, 10.55326060710041958 ) ) ;
#5030=CARTESIAN_POINT ( 'NONE',  ( 17.19109055900979399, 108.7710072034773532, -4.291528102762561581 ) ) ;
#5045=CARTESIAN_POINT ( 'NONE',  ( 40.68735894681399401, 154.1427111589966898, 9.763412716672732472 ) ) ;
#5050=CARTESIAN_POINT ( 'NONE',  ( 76.97600836722278927, 116.3222765712875031, 6.700797217583226661 ) ) ;
#5051=CARTESIAN_POINT ( 'NONE',  ( 22.10153057061799231, 100.9866247252079745, 1.346821830042071566 ) ) ;
#5063=CARTESIAN_POINT ( 'NONE',  ( 33.21234449867455396, 152.6251194638087725, -9.489586336475131390 ) ) ;
#5072=CARTESIAN_POINT ( 'NONE',  ( 57.14511974427749408, 88.72838517433189054, 6.862995836283489304 ) ) ;
#5080=CARTESIAN_POINT ( 'NONE',  ( 44.40591325931411859, 91.66001841764941105, -0.6336051400208910778 ) ) ;
#5091=CARTESIAN_POINT ( 'NONE',  ( 32.47916914626341622, 146.0660553311768979, 3.489959554161691013 ) ) ;
#5097=CARTESIAN_POINT ( 'NONE',  ( 38.76483609280177944, 144.5439415482201184, 31.56623162037504926 ) ) ;
#5103=CARTESIAN_POINT ( 'NONE',  ( 75.25890017065090376, 108.1762305904371004, -2.022566849933696620 ) ) ;
#5109=CARTESIAN_POINT ( 'NONE',  ( 10.61900875472251649, 108.8314319666055212, -5.279948415675857376 ) ) ;
#5111=CARTESIAN_POINT ( 'NONE',  ( 60.38095089740433252, 142.1228462996803046, -2.343495028824083004 ) ) ;
#5117=CARTESIAN_POINT ( 'NONE',  ( 62.47932545177000208, 147.9683691103492436, 5.510132816154444946 ) ) ;
#5127=CARTESIAN_POINT ( 'NONE',  ( 70.85748824340309682, 124.3570181999574515, -1.510321027129504889 ) ) ;
#5133=DIRECTION ( 'NONE',  ( 0.000000000000000000, 0.000000000000000000, 1.000000000000000000 ) ) ;
#5134=CARTESIAN_POINT ( 'NONE',  ( 10.16827731527805767, 110.2528774685086574, 8.767718578943870966 ) ) ;
#5136=CARTESIAN_POINT ( 'NONE',  ( 61.95829188091916961, 99.12855633088805973, 0.5892133286805102399 ) ) ;
#5150=CARTESIAN_POINT ( 'NONE',  ( 53.27251631713230040, 87.16359876908097704, 20.00146008344694337 ) ) ;
#5155=CARTESIAN_POINT ( 'NONE',  ( 74.11624783127615501, 105.8034190341144978, 7.057826790323951549 ) ) ;
#5156=CARTESIAN_POINT ( 'NONE',  ( 32.38101408406643600, 93.78751416920769657, -6.153149741203968404 ) ) ;
#5166=CARTESIAN_POINT ( 'NONE',  ( 74.95715479139145998, 107.8263973513541742, -14.01376907723217613 ) ) ;
#5178=CARTESIAN_POINT ( 'NONE',  ( 75.59501567365037999, 109.4093883240155378, 12.93430809701916750 ) ) ;
#5184=CARTESIAN_POINT ( 'NONE',  ( 43.42882498487155374, 148.1844126167958393, 2.937742163556189112 ) ) ;
#5198=CARTESIAN_POINT ( 'NONE',  ( 60.04598833032897431, 142.2798636455802921, -15.36278432740704147 ) ) ;
#5209=CARTESIAN_POINT ( 'NONE',  ( 31.20897972572539558, 148.4098837309084900, 17.43780275515693390 ) ) ;
#5213=CARTESIAN_POINT ( 'NONE',  ( 65.27013532398795803, 145.9152199903044504, 11.62486143609835310 ) ) ;
#5220=CARTESIAN_POINT ( 'NONE',  ( 76.92284642892752800, 124.5854180935290714, 5.434424407683230207 ) ) ;
#5222=CARTESIAN_POINT ( 'NONE',  ( 70.35668680342836012, 113.0167181193761508, -8.057780719902234878 ) ) ;
#5228=CARTESIAN_POINT ( 'NONE',  ( 52.64611633815218283, 152.6728927476294189, 5.153103026933554709 ) ) ;
#5235=CARTESIAN_POINT ( 'NONE',  ( 66.49460585200260709, 135.5194395740885511, -1.986604139701473759 ) ) ;
#5241=CARTESIAN_POINT ( 'NONE',  ( 68.01140435219951996, 119.9070776186055838, 50.00000000000002842 ) ) ;
#5244=CARTESIAN_POINT ( 'NONE',  ( 31.68064667488295783, 94.17100518331969283, -5.125072385659846574 ) ) ;
#5260=CARTESIAN_POINT ( 'NONE',  ( 48.82767110959031243, 147.5835523268705458, -3.847861628839052361 ) ) ;
#5265=CARTESIAN_POINT ( 'NONE',  ( 21.64910689156460322, 146.5545592879464607, 4.081561387450916456 ) ) ;
#5266=CARTESIAN_POINT ( 'NONE',  ( 41.15066532084431827, 91.76888749123396849, -6.510040445920065366 ) ) ;
#5286=CARTESIAN_POINT ( 'NONE',  ( 39.19820123626366382, 154.0079489008930693, -4.284297094604833767 ) ) ;
#5291=CARTESIAN_POINT ( 'NONE',  ( 60.26010703883354580, 142.3196469542212697, 3.652109145728902551 ) ) ;
#5300=EDGE_CURVE ( 'NONE', #19976, #8368, #20491, .T. ) ;
#5305=CARTESIAN_POINT ( 'NONE',  ( 23.31543935874208273, 139.7533899986231916, -16.95817871342526573 ) ) ;
#5309=CARTESIAN_POINT ( 'NONE',  ( 44.31278541401216842, 94.93890120144995137, 29.37189892749850273 ) ) ;
#5312=CARTESIAN_POINT ( 'NONE',  ( 39.70492769379191600, 144.6885458319320321, 37.97538637126935868 ) ) ;
#5317=CARTESIAN_POINT ( 'NONE',  ( 14.48810111090402941, 100.9784058478479523, 15.43442115621699529 ) ) ;
#5323=CARTESIAN_POINT ( 'NONE',  ( 11.39584491653312526, 106.7788786240791978, 8.648593811254444930 ) ) ;
#5325=CARTESIAN_POINT ( 'NONE',  ( 53.00431643774457768, 93.53749527547704190, -6.986323292181506162 ) ) ;
#5330=CARTESIAN_POINT ( 'NONE',  ( 69.27296957579615366, 97.94681810169329594, -0.6368323762655749842 ) ) ;
#5338=CARTESIAN_POINT ( 'NONE',  ( 64.30534519084480394, 138.3942263399134447, -9.129458798097310535 ) ) ;
#5348=CARTESIAN_POINT ( 'NONE',  ( 42.05360093099289287, 148.0107091728485500, 4.874927614337289938 ) ) ;
#5365=CARTESIAN_POINT ( 'NONE',  ( 39.80927132972225024, 148.0054509460111660, -4.205104553811644941 ) ) ;
#5370=CARTESIAN_POINT ( 'NONE',  ( 68.88151390383544026, 142.3271613368909811, -9.208263745312144977 ) ) ;
#5371=CARTESIAN_POINT ( 'NONE',  ( 63.85057544308668298, 100.9084186779620609, 13.48995955233852229 ) ) ;
#5380=CARTESIAN_POINT ( 'NONE',  ( 54.06307869441068448, 152.2224424482157303, -15.79932498977872868 ) ) ;
#5390=CARTESIAN_POINT ( 'NONE',  ( 77.07719282571002850, 116.5297446719512209, 12.69640610750513865 ) ) ;
#5395=CARTESIAN_POINT ( 'NONE',  ( 12.26432857192422432, 135.0705202968918570, 22.59931835930844457 ) ) ;
#5404=CARTESIAN_POINT ( 'NONE',  ( 70.51576897149806200, 126.1317638695992116, 12.41827883020830470 ) ) ;
#5406=CARTESIAN_POINT ( 'NONE',  ( 43.01140435219951996, 144.9070776186055696, 29.21067981925357060 ) ) ;
#5416=CARTESIAN_POINT ( 'NONE',  ( 19.13088699441526686, 95.37848931739559077, 15.19637875606281341 ) ) ;
#5422=CARTESIAN_POINT ( 'NONE',  ( 10.91571581598819662, 131.8149664739095783, 9.482090752819161139 ) ) ;
#5424=CARTESIAN_POINT ( 'NONE',  ( 70.74141321743030630, 114.7826485538520416, 5.870819564965037429 ) ) ;
#5430=CARTESIAN_POINT ( 'NONE',  ( 20.75180444880664510, 93.89949152720284076, -5.875022464008872625 ) ) ;
#5439=CARTESIAN_POINT ( 'NONE',  ( 70.84063976188440392, 115.3547488198113200, -1.153064885589385025 ) ) ;
#5449=CARTESIAN_POINT ( 'NONE',  ( 39.64555921537804295, 153.8934876517313342, -16.27550955686750456 ) ) ;
#5459=FACE_BOUND ( 'NONE', #3115, .T. ) ;
#5465=CARTESIAN_POINT ( 'NONE',  ( 19.22998607435487273, 95.16999353120945671, 21.19198650444592857 ) ) ;
#5470=CARTESIAN_POINT ( 'NONE',  ( 8.779377865064803999, 119.6051361893432130, -4.922546661887801100 ) ) ;
#5471=CARTESIAN_POINT ( 'NONE',  ( 56.80456144658707274, 95.31062238922963559, 13.84685026556700116 ) ) ;
#5481=CARTESIAN_POINT ( 'NONE',  ( 23.45433402446531446, 147.8217840461813068, -16.84717431919864339 ) ) ;
#5489=CARTESIAN_POINT ( 'NONE',  ( 72.33162239183086228, 137.5781058455011703, 11.98183203572534872 ) ) ;
#5495=CARTESIAN_POINT ( 'NONE',  ( 55.43026649837064213, 94.49908577724413306, 5.913859291446645905 ) ) ;
#5499=ORIENTED_EDGE ( 'NONE', *, *, #12715, .F. ) ;
#5506=CARTESIAN_POINT ( 'NONE',  ( 65.44800906011916197, 136.9904114405718758, 11.94221925691594777 ) ) ;
#5507=MECHANICAL_DESIGN_GEOMETRIC_PRESENTATION_REPRESENTATION('',(#2689),#15910);
#5511=CARTESIAN_POINT ( 'NONE',  ( 43.01140435219951996, 94.90707761860558378, 29.21067981925357060 ) ) ;
#5518=AXIS2_PLACEMENT_3D ( 'NONE', #21715, #19723, #2964 ) ;
#5519=CARTESIAN_POINT ( 'NONE',  ( 20.86407471411557779, 93.69780688484533471, 0.1205864258981524662 ) ) ;
#5525=CARTESIAN_POINT ( 'NONE',  ( 17.60877916486148465, 96.95950790538488206, 1.267834678905774393 ) ) ;
#5527=CARTESIAN_POINT ( 'NONE',  ( 14.82803154953497859, 120.8649872489531987, 9.204245268424362081 ) ) ;
#5535=CARTESIAN_POINT ( 'NONE',  ( 47.47886434171987702, 153.8471147930492862, -3.017879606865911502 ) ) ;
#5551=CARTESIAN_POINT ( 'NONE',  ( 70.48507635059884535, 125.9029633330538189, 6.422671151982867421 ) ) ;
#5571=CARTESIAN_POINT ( 'NONE',  ( 33.94330515458147346, 146.6952251797808628, -4.443226218224292978 ) ) ;
#5576=CARTESIAN_POINT ( 'NONE',  ( 23.17700876947760591, 147.8092992330439586, -3.851376987104358829 ) ) ;
#5577=CARTESIAN_POINT ( 'NONE',  ( 34.07414013685151843, 93.16113583794900421, 7.775673839875955728 ) ) ;
#5579=EDGE_CURVE ( 'NONE', #18715, #2680, #15868, .T. ) ;
#5588=CARTESIAN_POINT ( 'NONE',  ( 22.33864107606189719, 92.72021074822440312, 2.057911645927444244 ) ) ;
#5596=CARTESIAN_POINT ( 'NONE',  ( 9.822352152143091431, 128.2981216602131553, 9.363167623699879982 ) ) ;
#5604=CARTESIAN_POINT ( 'NONE',  ( 19.04663372520828801, 134.9227921665808765, 15.79488502079956547 ) ) ;
#5618=CARTESIAN_POINT ( 'NONE',  ( 39.35338560254503903, 91.94623120232463975, 14.56122079753911081 ) ) ;
#5630=CARTESIAN_POINT ( 'NONE',  ( 36.32848368193762667, 153.5644447507555981, 2.620555573812929584 ) ) ;
#5640=CARTESIAN_POINT ( 'NONE',  ( 67.71458430423905384, 106.3058120325361671, 6.227933542621733487 ) ) ;
#5648=CARTESIAN_POINT ( 'NONE',  ( 10.42839491720816625, 130.4056617841633283, -4.565575592310756825 ) ) ;
#5653=DIRECTION ( 'NONE',  ( 1.000000000000000000, 0.000000000000000000, 0.000000000000000000 ) ) ;
#5660=CARTESIAN_POINT ( 'NONE',  ( 76.79083979644461522, 114.3551126354810492, -1.232281421064668869 ) ) ;
#5666=CARTESIAN_POINT ( 'NONE',  ( 69.68093098098093208, 128.8215514297462789, 6.303499042945750475 ) ) ;
#5685=CARTESIAN_POINT ( 'NONE',  ( 37.19530960600651071, 92.23011878076297876, 13.65210914576621271 ) ) ;
#5691=CARTESIAN_POINT ( 'NONE',  ( 18.35401747797491723, 143.4883766228698221, 10.92869415326320670 ) ) ;
#5692=CARTESIAN_POINT ( 'NONE',  ( 17.98614708603287937, 106.9092867359673704, 15.63253669370310384 ) ) ;
#5694=CIRCLE ( 'NONE', #19426, 2.999999999999997780 ) ;
#5695=CIRCLE ( 'NONE', #17315, 24.99999999999999289 ) ;
#5703=CARTESIAN_POINT ( 'NONE',  ( 29.26409511065843105, 88.64202804534433255, -5.203872050689020590 ) ) ;
#5705=CARTESIAN_POINT ( 'NONE',  ( 76.40658810299491677, 127.4365358892444959, 12.33923360994393903 ) ) ;
#5711=CARTESIAN_POINT ( 'NONE',  ( 75.25890017065090376, 108.1762305904371004, -2.022566849933696620 ) ) ;
#5718=CARTESIAN_POINT ( 'NONE',  ( 16.98434641657835797, 108.8433182140206270, 14.72356627441054755 ) ) ;
#5729=CARTESIAN_POINT ( 'NONE',  ( 38.46765184765857981, 147.6574975633170936, -2.267929528491105629 ) ) ;
#5741=CARTESIAN_POINT ( 'NONE',  ( 75.01029411920679024, 107.5147569559006655, 5.001370044594233732 ) ) ;
#5748=CARTESIAN_POINT ( 'NONE',  ( 21.71662816054514167, 101.4213758857254675, 8.370706496969875232 ) ) ;
#5753=CARTESIAN_POINT ( 'NONE',  ( 26.13368487350976110, 90.12329638092472806, 0.9106621812756837686 ) ) ;
#5765=CARTESIAN_POINT ( 'NONE',  ( 71.86557814238962294, 101.4853659568252766, -7.779689512009451136 ) ) ;
#5771=CARTESIAN_POINT ( 'NONE',  ( 29.11053999216420252, 151.1052802516552163, -16.63225393015772724 ) ) ;
#5788=CARTESIAN_POINT ( 'NONE',  ( 22.35924357203464297, 139.2281224154095014, 9.009280560090923373 ) ) ;
#5794=CARTESIAN_POINT ( 'NONE',  ( 71.86557814238962294, 101.4853659568252766, -7.779689512009451136 ) ) ;
#5795=CARTESIAN_POINT ( 'NONE',  ( 70.74141321743030630, 114.7826485538520416, 5.870819564965037429 ) ) ;
#5804=CARTESIAN_POINT ( 'NONE',  ( 11.65896226128411683, 106.3627486108568547, -4.370744638174604013 ) ) ;
#5806=CARTESIAN_POINT ( 'NONE',  ( 45.29500579500201951, 154.0643053174194961, 10.91066218119221709 ) ) ;
#5812=CARTESIAN_POINT ( 'NONE',  ( 76.33227852969314142, 111.7084249013780806, -2.141487123205697340 ) ) ;
#5818=CARTESIAN_POINT ( 'NONE',  ( 29.27693512915957541, 95.18479568265063051, 6.985315079919499404 ) ) ;
#5829=CARTESIAN_POINT ( 'NONE',  ( 46.87248680087107999, 147.7605717807558676, -8.934501345478663481 ) ) ;
#5839=CARTESIAN_POINT ( 'NONE',  ( 77.15313604554262383, 122.4041478163663612, -8.494263314424808087 ) ) ;
#5847=CARTESIAN_POINT ( 'NONE',  ( 13.73412108254838238, 102.0109333093626134, 0.4776103675054816922 ) ) ;
#5848=VERTEX_POINT ( 'NONE', #13627 ) ;
#5855=CARTESIAN_POINT ( 'NONE',  ( 17.48807464456866256, 131.8965856249792523, 2.656420782620954935 ) ) ;
#5864=CARTESIAN_POINT ( 'NONE',  ( 14.15704070161504369, 138.3271338521546454, 9.720138693322796897 ) ) ;
#5865=CARTESIAN_POINT ( 'NONE',  ( 38.01123955261142129, 95.41221383034442738, 34.53828804502999361 ) ) ;
#5873=CARTESIAN_POINT ( 'NONE',  ( 71.53613896966024299, 138.8348963267899592, -2.065403804986401859 ) ) ;
#5897=CARTESIAN_POINT ( 'NONE',  ( 62.98455118117477980, 139.9299249275418617, 10.79496628861178387 ) ) ;
#5900=CIRCLE ( 'NONE', #2384, 10.00000000000000888 ) ;
#5902=ORIENTED_EDGE ( 'NONE', *, *, #18492, .T. ) ;
#5904=CARTESIAN_POINT ( 'NONE',  ( 43.80529445460960858, 154.1304981347762748, -3.137004163733609907 ) ) ;
#5905=CARTESIAN_POINT ( 'NONE',  ( 24.58042389364637259, 98.66975071380154816, -11.79164420265881574 ) ) ;
#5916=CARTESIAN_POINT ( 'NONE',  ( 11.06625761453251933, 131.9899775861109106, 3.486483074593720755 ) ) ;
#5919=CARTESIAN_POINT ( 'NONE',  ( 9.976645104453018220, 110.9295780357170571, 15.79146183154218619 ) ) ;
#5921=DIRECTION ( 'NONE',  ( -0.3428981916074304581, 0.9393725726208712601, 0.000000000000000000 ) ) ;
#5924=CARTESIAN_POINT ( 'NONE',  ( 76.06694498870253085, 129.1134374410657983, 4.287174360044270216 ) ) ;
#5930=CARTESIAN_POINT ( 'NONE',  ( 37.19530960600651071, 92.23011878076297876, 13.65210914576621271 ) ) ;
#5941=CARTESIAN_POINT ( 'NONE',  ( 31.68064667488295783, 94.17100518331969283, -5.125072385659846574 ) ) ;
#5956=CARTESIAN_POINT ( 'NONE',  ( 20.33033954036769941, 94.15838586645493535, 7.144317217164116052 ) ) ;
#5964=CARTESIAN_POINT ( 'NONE',  ( 19.52755003174225124, 104.2962547294809070, 15.51356631106660089 ) ) ;
#5971=CARTESIAN_POINT ( 'NONE',  ( 34.41316853928974950, 153.0433231119815503, 10.55326060710041958 ) ) ;
#5972=CARTESIAN_POINT ( 'NONE',  ( 40.78964507673602924, 95.00417210663486856, 38.70176206714167932 ) ) ;
#5982=CARTESIAN_POINT ( 'NONE',  ( 73.40451243997107156, 135.6611253642151098, -1.946480675884423084 ) ) ;
#5990=ORIENTED_EDGE ( 'NONE', *, *, #1181, .T. ) ;
#6005=CARTESIAN_POINT ( 'NONE',  ( 70.99289463508769416, 124.0080672713295087, 11.50917073501047483 ) ) ;
#6011=CARTESIAN_POINT ( 'NONE',  ( 42.92180000979148957, 85.67454126555050209, 7.339147150375312734 ) ) ;
#6012=CARTESIAN_POINT ( 'NONE',  ( 26.96882349746146446, 96.81297435472995971, -11.91061488385382106 ) ) ;
#6013=CARTESIAN_POINT ( 'NONE',  ( 28.88048086162541850, 151.0887240815949895, -10.63664014359656385 ) ) ;
#6022=CARTESIAN_POINT ( 'NONE',  ( 58.73109577922829061, 150.2274887891485662, -1.632724326791204605 ) ) ;
#6024=CARTESIAN_POINT ( 'NONE',  ( 41.61242760320212852, 154.1118385459532760, 10.79173905232880237 ) ) ;
#6030=CARTESIAN_POINT ( 'NONE',  ( 13.73412108254838238, 102.0109333093626134, 0.4776103675054816922 ) ) ;
#6037=CARTESIAN_POINT ( 'NONE',  ( 42.59292608294269655, 91.62918162712271908, 20.43785202907404752 ) ) ;
#6051=CARTESIAN_POINT ( 'NONE',  ( 15.53781593631592983, 113.9137188375014347, -11.07707013084618097 ) ) ;
#6059=CARTESIAN_POINT ( 'NONE',  ( 54.54805624998882507, 152.1374805055981199, -2.779977617235711129 ) ) ;
#6066=CARTESIAN_POINT ( 'NONE',  ( 8.804574439154260190, 117.1883747968346654, 15.00137004459121393 ) ) ;
#6073=CARTESIAN_POINT ( 'NONE',  ( 48.35156950851215640, 92.21792820573091376, 14.20396468032920012 ) ) ;
#6081=CARTESIAN_POINT ( 'NONE',  ( 38.04450641318627646, 95.40535984405393322, 33.55020052675506292 ) ) ;
#6088=CARTESIAN_POINT ( 'NONE',  ( 23.67598417054553295, 91.65793073385727041, -5.994147020910363999 ) ) ;
#6111=CARTESIAN_POINT ( 'NONE',  ( 32.01435502045076475, 93.85226834503447435, 6.866149820358673495 ) ) ;
#6117=CARTESIAN_POINT ( 'NONE',  ( 61.76154402333882132, 148.5480768402654803, 4.482004293238171400 ) ) ;
#6118=CARTESIAN_POINT ( 'NONE',  ( 55.45346087869361185, 145.1240540049360845, -8.577242388453932165 ) ) ;
#6119=CARTESIAN_POINT ( 'NONE',  ( 54.54805624998882507, 152.1374805055981199, -2.779977617235711129 ) ) ;
#6128=CARTESIAN_POINT ( 'NONE',  ( 16.16624775068580533, 140.9673012293996237, 10.82561872270659009 ) ) ;
#6132=CARTESIAN_POINT ( 'NONE',  ( 49.46632042442519861, 86.28835692931116341, 14.12497754236212977 ) ) ;
#6137=CARTESIAN_POINT ( 'NONE',  ( 26.28242620001017471, 89.94675250444232972, 6.906269859504051922 ) ) ;
#6142=CARTESIAN_POINT ( 'NONE',  ( 24.78883071187807730, 141.3519591882296709, -10.86778418981948846 ) ) ;
#6145=ORIENTED_EDGE ( 'NONE', *, *, #11081, .T. ) ;
#6152=CARTESIAN_POINT ( 'NONE',  ( 61.44294336830710535, 141.1433446673695471, 5.708471897238777792 ) ) ;
#6154=CARTESIAN_POINT ( 'NONE',  ( 47.75558613178728251, 144.4531355194695550, 35.82300994916138848 ) ) ;
#6161=CARTESIAN_POINT ( 'NONE',  ( 68.88151390383544026, 142.3271613368909811, -9.208263745312144977 ) ) ;
#6170=CARTESIAN_POINT ( 'NONE',  ( 53.27251631713230040, 87.16359876908097704, 20.00146008344694337 ) ) ;
#6174=CARTESIAN_POINT ( 'NONE',  ( 61.38527826276358468, 91.11739401521901982, -13.29920278214092200 ) ) ;
#6179=CARTESIAN_POINT ( 'NONE',  ( 61.33076419740685736, 141.3451534613812441, 11.70407797152743079 ) ) ;
#6187=CARTESIAN_POINT ( 'NONE',  ( 61.76154402333882132, 148.5480768402654803, 4.482004293238171400 ) ) ;
#6197=CARTESIAN_POINT ( 'NONE',  ( 66.24914683137549787, 94.76885710642066840, 6.506024766557033878 ) ) ;
#6207=CARTESIAN_POINT ( 'NONE',  ( 23.10700517764655260, 139.6571016847272801, -10.96257334342637435 ) ) ;
#6223=CARTESIAN_POINT ( 'NONE',  ( 51.94691807752363388, 146.6530262932614050, -9.724486432582017059 ) ) ;
#6230=CARTESIAN_POINT ( 'NONE',  ( 66.76198117565915879, 95.25264312590786631, -0.5179092472497510702 ) ) ;
#6231=CARTESIAN_POINT ( 'NONE',  ( 64.82873087846098770, 102.1656695083886603, -13.57732884656604355 ) ) ;
#6250=CARTESIAN_POINT ( 'NONE',  ( 8.804574439154260190, 117.1883747968346654, 15.00137004459121393 ) ) ;
#6256=CARTESIAN_POINT ( 'NONE',  ( 58.35211712195835076, 96.24552883246097679, -7.224606741634919338 ) ) ;
#6266=CARTESIAN_POINT ( 'NONE',  ( 36.80677928932056631, 92.47987693618573246, 1.660900796654692702 ) ) ;
#6277=CARTESIAN_POINT ( 'NONE',  ( 74.62708615766334219, 133.0342049366344384, -8.851289726714327344 ) ) ;
#6286=CARTESIAN_POINT ( 'NONE',  ( 9.955767346236717330, 110.6995739201198887, 21.78706596723887756 ) ) ;
#6289=CARTESIAN_POINT ( 'NONE',  ( 13.96574040630659752, 137.8735611475157157, -3.299202782472894224 ) ) ;
#6292=CARTESIAN_POINT ( 'NONE',  ( 68.77576173894735234, 108.4446202281264249, 13.13264940013829296 ) ) ;
#6295=DIRECTION ( 'NONE',  ( -0.000000000000000000, 1.000000000000000000, -0.000000000000000000 ) ) ;
#6299=CARTESIAN_POINT ( 'NONE',  ( 71.19791805076843616, 120.7596060772701776, 5.632536115698772328 ) ) ;
#6302=CARTESIAN_POINT ( 'NONE',  ( 74.27779736592162863, 105.9683817680885056, 13.05343286460986363 ) ) ;
#6307=CARTESIAN_POINT ( 'NONE',  ( 41.39629556124358345, 144.8566973352396587, 38.95396702123350252 ) ) ;
#6313=CARTESIAN_POINT ( 'NONE',  ( 13.78455932396994577, 137.7305411390292420, 2.696406107442721467 ) ) ;
#6337=CARTESIAN_POINT ( 'NONE',  ( 21.79768317403592803, 101.2052074350461339, 14.36631359211887649 ) ) ;
#6343=CARTESIAN_POINT ( 'NONE',  ( 73.40451243997107156, 135.6611253642151098, -1.946480675884423084 ) ) ;
#6344=CARTESIAN_POINT ( 'NONE',  ( 49.88381083390898851, 92.64041853056629350, -12.86295667411130239 ) ) ;
#6363=CARTESIAN_POINT ( 'NONE',  ( 58.41865009756546812, 150.5677012977470781, 10.35848337793017393 ) ) ;
#6369=CARTESIAN_POINT ( 'NONE',  ( 64.05606230151549596, 101.0139342820504993, 19.48556066606253978 ) ) ;
#6372=DIRECTION ( 'NONE',  ( -1.000000000000000000, 0.000000000000000000, -0.000000000000000000 ) ) ;
#6373=ORIENTED_EDGE ( 'NONE', *, *, #19599, .T. ) ;
#6378=CARTESIAN_POINT ( 'NONE',  ( 59.14563986918259531, 96.87627350248034475, 7.732070471200789719 ) ) ;
#6391=CARTESIAN_POINT ( 'NONE',  ( 9.021810916323596885, 123.9851095102452945, 2.220310480865780534 ) ) ;
#6397=CARTESIAN_POINT ( 'NONE',  ( 49.69400319086401652, 86.25038505451357196, 20.12058643263999969 ) ) ;
#6400=CARTESIAN_POINT ( 'NONE',  ( 9.783399875253829592, 127.8057224500684015, -3.656374068424393275 ) ) ;
#6405=CARTESIAN_POINT ( 'NONE',  ( 16.70103016558074316, 129.9804388327498827, 16.57432765154378629 ) ) ;
#6408=LINE ( 'NONE', #8183, #19940 ) ;
#6413=CARTESIAN_POINT ( 'NONE',  ( 42.95897134029118547, 91.70801217734280897, 7.418363685804686192 ) ) ;
#6425=CARTESIAN_POINT ( 'NONE',  ( 25.52397925108762067, 90.47728371212039633, 7.934596195134201224 ) ) ;
#6434=ORIENTED_EDGE ( 'NONE', *, *, #12395, .F. ) ;
#6449=CARTESIAN_POINT ( 'NONE',  ( 14.76087776054169787, 121.2312262212812755, 22.22355758277721804 ) ) ;
#6457=CARTESIAN_POINT ( 'NONE',  ( 42.74273477336613780, 91.78896094402264794, 1.422757611514577247 ) ) ;
#6474=CARTESIAN_POINT ( 'NONE',  ( 8.710246811478747020, 120.8788544656517274, 15.12029029225770316 ) ) ;
#6480=CARTESIAN_POINT ( 'NONE',  ( 56.11190468687431832, 151.4478768383145280, 5.272225788895710252 ) ) ;
#6481=CARTESIAN_POINT ( 'NONE',  ( 71.28758990370504023, 120.3962046462169440, 18.65202787790538608 ) ) ;
#6492=CARTESIAN_POINT ( 'NONE',  ( 19.41497643977705323, 135.2012136132025546, 3.803670830490076149 ) ) ;
#6504=CARTESIAN_POINT ( 'NONE',  ( 13.78455932396994577, 137.7305411390292420, 2.696406107442721467 ) ) ;
#6512=CARTESIAN_POINT ( 'NONE',  ( 8.710246811478747020, 120.8788544656517274, 15.12029029225770316 ) ) ;
#6515=CARTESIAN_POINT ( 'NONE',  ( 40.51949181395973199, 85.84442682937354618, -12.58519764931165241 ) ) ;
#6517=ORIENTED_EDGE ( 'NONE', *, *, #14589, .F. ) ;
#6525=CARTESIAN_POINT ( 'NONE',  ( 59.83664469576316236, 97.27638873328486113, 6.703993115985443119 ) ) ;
#6528=CARTESIAN_POINT ( 'NONE',  ( 12.61881386508366809, 104.1535352963828984, 15.55354899318430739 ) ) ;
#6538=CARTESIAN_POINT ( 'NONE',  ( 9.468627745026951814, 113.0646104733145592, 1.862908727141013854 ) ) ;
#6543=CARTESIAN_POINT ( 'NONE',  ( 71.14040157825178312, 139.4183699182763974, -9.089337262093875935 ) ) ;
#6547=CARTESIAN_POINT ( 'NONE',  ( 66.16974147772015158, 135.9983230778657344, -9.010293137571032673 ) ) ;
#6552=CARTESIAN_POINT ( 'NONE',  ( 32.31036143884366396, 152.4250368413922274, -10.51794503956956817 ) ) ;
#6567=CARTESIAN_POINT ( 'NONE',  ( 20.79828168028384994, 137.4105449198869735, 15.91385929137521771 ) ) ;
#6574=CARTESIAN_POINT ( 'NONE',  ( 9.203281625063985061, 114.5318647093721864, 15.91056058043385413 ) ) ;
#6576=CARTESIAN_POINT ( 'NONE',  ( 55.97020510223934764, 144.8627979930266463, -1.553355716038981038 ) ) ;
#6594=CARTESIAN_POINT ( 'NONE',  ( 14.94030450088465400, 100.1727563578744196, 14.40630071170483362 ) ) ;
#6599=CARTESIAN_POINT ( 'NONE',  ( 25.37887452999470028, 90.65668055682171200, 1.938985092122112563 ) ) ;
#6600=CARTESIAN_POINT ( 'NONE',  ( 22.56676867748217674, 139.3294883087844198, 3.013676707730225779 ) ) ;
#6614=CARTESIAN_POINT ( 'NONE',  ( 45.08035905667198762, 147.9511986603014861, 4.994099723559113357 ) ) ;
#6624=CARTESIAN_POINT ( 'NONE',  ( 57.78275410301085913, 89.02518083909171764, -0.1607367497116551913 ) ) ;
#6633=CARTESIAN_POINT ( 'NONE',  ( 42.84661501159713026, 148.1872198635363134, -4.086158671962061284 ) ) ;
#6639=CARTESIAN_POINT ( 'NONE',  ( 12.20328755962376199, 134.6477104347696923, -3.418325544530929516 ) ) ;
#6648=CARTESIAN_POINT ( 'NONE',  ( 50.21395344324809429, 147.1711500555979626, 4.203964687196366512 ) ) ;
#6656=CARTESIAN_POINT ( 'NONE',  ( 39.24377615895817684, 144.6226614538730928, 30.90720150815158718 ) ) ;
#6662=CARTESIAN_POINT ( 'NONE',  ( 63.41425016244589585, 92.41789933959738335, 6.624947895572852019 ) ) ;
#6668=CARTESIAN_POINT ( 'NONE',  ( 64.59149290518072917, 93.33317027722591774, -7.422718449586769296 ) ) ;
#6670=PRESENTATION_STYLE_ASSIGNMENT (( #6879 ) ) ;
#6675=CARTESIAN_POINT ( 'NONE',  ( 68.88151390383544026, 142.3271613368909811, -9.208263745312144977 ) ) ;
#6686=CARTESIAN_POINT ( 'NONE',  ( 28.77282558494574971, 95.47244942437217219, 14.00900696324737282 ) ) ;
#6693=CARTESIAN_POINT ( 'NONE',  ( 10.91571581598819662, 131.8149664739095783, 9.482090752819161139 ) ) ;
#6695=CARTESIAN_POINT ( 'NONE',  ( 15.97902590142590462, 112.1642626292039324, 2.851329040111875823 ) ) ;
#6711=CARTESIAN_POINT ( 'NONE',  ( 32.32016755483360271, 87.30015788337030358, 13.69171886368053492 ) ) ;
#6717=CARTESIAN_POINT ( 'NONE',  ( 8.886384673113061794, 121.3059481585812733, 3.129088064915290346 ) ) ;
#6718=CARTESIAN_POINT ( 'NONE',  ( 64.66009251794113766, 101.8366349233107684, -0.5580327111990067701 ) ) ;
#6729=CARTESIAN_POINT ( 'NONE',  ( 61.38527826276358468, 91.11739401521901982, -13.29920278214092200 ) ) ;
#6735=DIRECTION ( 'NONE',  ( 0.9387810623359076345, 0.3426822732243071656, 0.03548206049944094970 ) ) ;
#6739=CARTESIAN_POINT ( 'NONE',  ( 76.04618105687035268, 128.8835079444423286, -1.708432735116285350 ) ) ;
#6746=CARTESIAN_POINT ( 'NONE',  ( 61.02373258766779429, 98.10483126312279012, -1.347972122102980119 ) ) ;
#6757=CARTESIAN_POINT ( 'NONE',  ( 16.56453993303484395, 129.6948329502664308, 9.561135973024818213 ) ) ;
#6759=CARTESIAN_POINT ( 'NONE',  ( 12.43312601512511151, 135.2277911470865490, 16.60371454366222466 ) ) ;
#6760=CARTESIAN_POINT ( 'NONE',  ( 43.01140435219951996, 70.71049967264875136, 39.21067981925356349 ) ) ;
#6768=CARTESIAN_POINT ( 'NONE',  ( 55.94180145820917716, 151.6039095241057453, 11.26783467880839140 ) ) ;
#6775=CARTESIAN_POINT ( 'NONE',  ( 43.01140435219951996, 119.9070776186055838, -19.99999999999998579 ) ) ;
#6779=CARTESIAN_POINT ( 'NONE',  ( 46.66836841558743032, 147.8683539324387368, -2.938892455568735240 ) ) ;
#6784=CARTESIAN_POINT ( 'NONE',  ( 21.64910689156460322, 146.5545592879464607, 4.081561387450916456 ) ) ;
#6795=CARTESIAN_POINT ( 'NONE',  ( 57.39747520560054284, 144.1616143014069280, -9.486357586414486676 ) ) ;
#6801=CARTESIAN_POINT ( 'NONE',  ( 70.62757080055673953, 99.67629488849819097, 13.29148015538516425 ) ) ;
#6802=CARTESIAN_POINT ( 'NONE',  ( 58.57598713290192904, 143.3259681031794059, -1.434385245616870197 ) ) ;
#6812=EDGE_CURVE ( 'NONE', #21236, #2680, #3254, .T. ) ;
#6818=CARTESIAN_POINT ( 'NONE',  ( 15.77498628565902727, 140.7233915340666499, 22.81684008552556975 ) ) ;
#6820=CARTESIAN_POINT ( 'NONE',  ( 46.37776046713125311, 85.92026137128108587, 1.224418530371263580 ) ) ;
#6821=CARTESIAN_POINT ( 'NONE',  ( 41.25620118372704326, 148.0523446076144580, 3.846850258842608117 ) ) ;
#6832=CARTESIAN_POINT ( 'NONE',  ( 74.63589561985200760, 132.8035080205385157, -14.84689682711585768 ) ) ;
#6841=CARTESIAN_POINT ( 'NONE',  ( 75.16956835342354282, 131.6452004531123805, 5.196376467030073165 ) ) ;
#6847=CARTESIAN_POINT ( 'NONE',  ( 28.99223550982291897, 144.4690685518502846, 2.342703524990218611 ) ) ;
#6857=CARTESIAN_POINT ( 'NONE',  ( 49.21618705061847265, 147.3337112213800140, -15.83906960951095577 ) ) ;
#6865=CARTESIAN_POINT ( 'NONE',  ( 41.39828712335587113, 144.8568216812500680, 29.46674713776155130 ) ) ;
#6870=CARTESIAN_POINT ( 'NONE',  ( 44.63232748576950115, 85.63068390643836381, -0.7129156696548789585 ) ) ;
#6877=CARTESIAN_POINT ( 'NONE',  ( 26.90790578767411390, 150.1165885900122987, 3.291480155758420345 ) ) ;
#6879=SURFACE_STYLE_USAGE ( .BOTH. , #17993 ) ;
#6886=CARTESIAN_POINT ( 'NONE',  ( 24.63684302007652249, 148.6959638282970957, 4.200683933265449532 ) ) ;
#6896=CARTESIAN_POINT ( 'NONE',  ( 43.64334309031418968, 148.0990856179656419, -3.057864931601543823 ) ) ;
#6905=CARTESIAN_POINT ( 'NONE',  ( 65.91867393726404600, 103.5983250578868109, 0.3515012976045437387 ) ) ;
#6922=CARTESIAN_POINT ( 'NONE',  ( 12.64719099284060988, 103.9244585094960769, 21.54915782717631600 ) ) ;
#6926=CARTESIAN_POINT ( 'NONE',  ( 37.47668497174467461, 153.6095807538456199, -2.346729193546184700 ) ) ;
#6928=CARTESIAN_POINT ( 'NONE',  ( 18.86999673272213229, 105.3337293714367604, -5.438779171309367833 ) ) ;
#6939=CARTESIAN_POINT ( 'NONE',  ( 68.96269327682742301, 142.1111764150114993, -15.20387477620461425 ) ) ;
#6949=CARTESIAN_POINT ( 'NONE',  ( 28.65042173108665935, 151.0721679115347911, -4.641026357035400451 ) ) ;
#6955=CARTESIAN_POINT ( 'NONE',  ( 48.82767110959031243, 147.5835523268705458, -3.847861628839052361 ) ) ;
#6956=FILL_AREA_STYLE ('',( #8394 ) ) ;
#6968=CARTESIAN_POINT ( 'NONE',  ( 22.52008984372607614, 139.2495111981779985, 17.01435058386764965 ) ) ;
#6977=CARTESIAN_POINT ( 'NONE',  ( 38.04401232081008288, 144.4086955619317507, 33.55330648861601617 ) ) ;
#6983=CARTESIAN_POINT ( 'NONE',  ( 18.14018356548558941, 143.3940520581896862, 16.92415443696469879 ) ) ;
#6989=CARTESIAN_POINT ( 'NONE',  ( 13.78455932396994577, 137.7305411390292420, 2.696406107442721467 ) ) ;
#6997=CARTESIAN_POINT ( 'NONE',  ( 43.80529445460960858, 154.1304981347762748, -3.137004163733609907 ) ) ;
#7006=CARTESIAN_POINT ( 'NONE',  ( 71.16904767199986281, 118.3707548728134213, -1.272037577920760665 ) ) ;
#7015=CARTESIAN_POINT ( 'NONE',  ( 42.16380956469475194, 91.80013758078052888, 8.446644326836734606 ) ) ;
#7025=DIRECTION ( 'NONE',  ( -0.000000000000000000, -0.000000000000000000, -1.000000000000000000 ) ) ;
#7030=CARTESIAN_POINT ( 'NONE',  ( 18.91286941000743838, 105.1068529970173699, 0.5568269029779387980 ) ) ;
#7034=CARTESIAN_POINT ( 'NONE',  ( 60.49690154327523572, 149.3382625450468311, -9.565656633516235630 ) ) ;
#7035=CARTESIAN_POINT ( 'NONE',  ( 15.38454125381035098, 114.2504036285165654, 1.942219256913226388 ) ) ;
#7045=CARTESIAN_POINT ( 'NONE',  ( 32.54106024366770811, 152.4163610972421452, -16.51355214031335805 ) ) ;
#7050=DIRECTION ( 'NONE',  ( 0.000000000000000000, 0.000000000000000000, 1.000000000000000000 ) ) ;
#7056=CARTESIAN_POINT ( 'NONE',  ( 53.70366401737062034, 152.5123965792994625, -3.808113302951443568 ) ) ;
#7061=CARTESIAN_POINT ( 'NONE',  ( 17.08493018425929932, 131.2036312357472241, 1.628145005703640624 ) ) ;
#7075=CARTESIAN_POINT ( 'NONE',  ( 58.12682455153977656, 96.19528378222683784, -13.22021563155647428 ) ) ;
#7081=CARTESIAN_POINT ( 'NONE',  ( 46.06263289999436239, 95.09248412622439162, 30.23627618186981536 ) ) ;
#7087=CARTESIAN_POINT ( 'NONE',  ( 53.04203944364535772, 87.17698241397053494, 14.00585298808814194 ) ) ;
#7093=CARTESIAN_POINT ( 'NONE',  ( 8.798315742295939046, 121.0924013121165075, 9.124689178586496752 ) ) ;
#7096=CARTESIAN_POINT ( 'NONE',  ( 71.19791805076843616, 120.7596060772701776, 5.632536115698772328 ) ) ;
#7104=CARTESIAN_POINT ( 'NONE',  ( 17.60877916486148465, 96.95950790538488206, 1.267834678905774393 ) ) ;
#7111=CARTESIAN_POINT ( 'NONE',  ( 44.18632541912793243, 91.73153706005567187, -6.629209314582290347 ) ) ;
#7120=CARTESIAN_POINT ( 'NONE',  ( 69.71546013739904879, 111.0973159356150717, 7.018072855358342466 ) ) ;
#7139=CARTESIAN_POINT ( 'NONE',  ( 9.157865646370469292, 114.3054763464604662, 21.90616645148510599 ) ) ;
#7145=CARTESIAN_POINT ( 'NONE',  ( 20.91437931538276374, 145.9617080342048894, -10.94665030085253044 ) ) ;
#7146=CARTESIAN_POINT ( 'NONE',  ( 42.95897134029118547, 91.70801217734280897, 7.418363685804686192 ) ) ;
#7155=CARTESIAN_POINT ( 'NONE',  ( 32.43765954726634959, 145.6647664193251615, 11.44158087452429129 ) ) ;
#7165=CARTESIAN_POINT ( 'NONE',  ( 71.08298874133512868, 139.6419663798271529, -3.093729572736475752 ) ) ;
#7170=CARTESIAN_POINT ( 'NONE',  ( 37.76446383830448639, 92.11682557054228937, 6.628417810721723313 ) ) ;
#7180=CARTESIAN_POINT ( 'NONE',  ( 70.04389262751028866, 127.6510855156269599, -14.64878692017946626 ) ) ;
#7183=CARTESIAN_POINT ( 'NONE',  ( 45.65510909715900567, 144.7672780766941401, 29.96360841760569116 ) ) ;
#7186=CARTESIAN_POINT ( 'NONE',  ( 47.25797261159726759, 95.27021368899106335, 31.56623162037505637 ) ) ;
#7194=CARTESIAN_POINT ( 'NONE',  ( 75.59501567365037999, 109.4093883240155378, 12.93430809701916750 ) ) ;
#7200=CARTESIAN_POINT ( 'NONE',  ( 76.79083979644461522, 114.3551126354810492, -1.232281421064668869 ) ) ;
#7202=CARTESIAN_POINT ( 'NONE',  ( 68.03731475862628031, 132.9047928164914367, -1.867435455408581912 ) ) ;
#7213=CARTESIAN_POINT ( 'NONE',  ( 11.67247064774405452, 106.1322524520788875, 1.624861436118421043 ) ) ;
#7231=CARTESIAN_POINT ( 'NONE',  ( 76.07019559177007295, 111.3280993686123281, -14.13269547130637704 ) ) ;
#7249=CARTESIAN_POINT ( 'NONE',  ( 31.11878897118147336, 145.5659923423516773, -4.562434011626001151 ) ) ;
#7254=CARTESIAN_POINT ( 'NONE',  ( 11.74529739132928619, 133.8467647624810581, -4.446451035385589279 ) ) ;
#7255=CARTESIAN_POINT ( 'NONE',  ( 35.91077447413180579, 147.1981228300969633, 10.63281669705329691 ) ) ;
#7256=PLANE ( 'NONE',  #12855 ) ;
#7260=B_SPLINE_CURVE_WITH_KNOTS ( 'NONE', 3,
 ( #6207, #20430, #1585, #13377, #16891, #15023, #10295, #1805, #15250, #148, #5005, #4888, #6547, #20324, #18337, #16786, #8640, #5222, #11609, #11938, #15362, #253, #18666, #5325, #10403, #16673, #12042, #13270, #18772, #17103, #18560, #20005, #18450, #1698, #2019, #8427, #21763, #3239, #8750, #9970, #8315, #20114, #11715, #3349, #15136, #39, #6779, #13486, #20218, #5111, #11828, #17321, #7202, #19203, #12362, #15879, #2441, #2231, #793, #8859, #12585, #7527, #15668, #19309, #14228, #9182, #18988, #9071, #20968, #10723, #15566, #20859, #7315, #8961, #10511, #14016, #12256, #5855, #10834, #4100, #9287, #4206, #571, #10935, #469, #17643, #368, #19101, #2550, #20751, #13801, #13905, #14120, #3891, #7096, #5424, #685, #5640, #2333, #3998, #15779, #10614, #20538, #17532, #12141, #17425, #18875, #3782, #7421, #5748, #17208, #2123, #20644, #12472, #5527, #13024, #21082, #4310, #14665, #19412, #18193, #11034, #17749, #9395, #1336, #19744, #4639, #2652, #6179, #11464, #19856, #4744, #7749, #11357, #18080, #2986, #6292, #3100, #16100, #9725, #15987, #11143, #6073, #16424, #898, #1012, #8069, #1119, #16316, #5964, #14776, #12690, #21518, #1226, #7639, #6405, #14555, #7853, #13130, #14341, #14448, #21185 ),
 .UNSPECIFIED., .F., .F.,
 ( 4, 2, 2, 2, 2, 2, 2, 2, 2, 2, 2, 2, 2, 2, 2, 2, 2, 2, 2, 2, 2, 2, 2, 2, 2, 2, 2, 2, 2, 2, 2, 2, 2, 2, 2, 2, 2, 2, 2, 2, 2, 2, 2, 2, 2, 2, 2, 2, 2, 2, 2, 2, 2, 2, 2, 2, 2, 2, 2, 2, 2, 2, 2, 2, 2, 2, 2, 2, 2, 2, 2, 2, 2, 2, 2, 2, 2, 2, 2, 2, 4 ),
 ( 0.000000000000000000, 0.008318061648474830982, 0.01871563870907547167, 0.02911321576967611582, 0.03951079283027675998, 0.04990836989087740067, 0.06030594695147804829, 0.07070352401207868898, 0.08110110107267932966, 0.09149867813327997035, 0.1018962551938806110, 0.1122938322544812378, 0.1226914093150818785, 0.1330889863756825053, 0.1434865634362831321, 0.1538841404968837590, 0.1642817175574844135, 0.1746792946180850126, 0.1850768716786856394, 0.1954744487392862939, 0.2058720257998869485, 0.2162696028604875753, 0.2266671799210882021, 0.2370647569816888289, 0.2474623340422894557, 0.2578599111028900825, 0.2682574881634907094, 0.2786550652240913362, 0.2890526422846919630, 0.2994502193452925343, 0.3098477964058931611, 0.3202453734664938434, 0.3306429505270944147, 0.3410405275876950415, 0.3514381046482956683, 0.3618356817088962951, 0.3722332587694969219, 0.3826308358300975487, 0.3930284128906983421, 0.4034259899512990799, 0.4138235670118998732, 0.4242211440725006666, 0.4346187211331003497, 0.4450162981936999218, 0.4554138752542995494, 0.4658114523148991770, 0.4762090293755007475, 0.4866066064361022070, 0.4970041834967036110, 0.5074017605573051259, 0.5177993376179057528, 0.5281969146785063796, 0.5385944917391070064, 0.5489920687997077442, 0.5593896458603083710, 0.5697872229209089978, 0.5801847999815096246, 0.5905823770421102514, 0.6009799541027108782, 0.6113775311633115050, 0.6217751082239121319, 0.6321726852845127587, 0.6425702623451133855, 0.6529678394057140123, 0.6633654164663146391, 0.6737629935269153769, 0.6841605705875142274, 0.6945581476481129668, 0.7049557247087120393, 0.7153533017693110008, 0.7257508788299132929, 0.7361484558905155851, 0.7465460329511179882, 0.7569436100117202804, 0.7673411870723210182, 0.7777387641329215340, 0.7881363411935222718, 0.7985339182541228986, 0.8080132075800156022, 0.8174924969059083057, 0.8280181261579530050 ),
 .UNSPECIFIED. ) ;
#7264=CARTESIAN_POINT ( 'NONE',  ( 73.15003751907750029, 103.8404476760371864, -6.870911935119222491 ) ) ;
#7273=CARTESIAN_POINT ( 'NONE',  ( 8.798315742295939046, 121.0924013121165075, 9.124689178586496752 ) ) ;
#7280=CARTESIAN_POINT ( 'NONE',  ( 31.20897972572456069, 148.4098837309091721, 17.43780275515692679 ) ) ;
#7282=CARTESIAN_POINT ( 'NONE',  ( 68.16012629694054681, 106.9699110742356396, 5.199846382127304878 ) ) ;
#7295=CARTESIAN_POINT ( 'NONE',  ( 15.80414578680225723, 112.4924633436790344, 15.87081086175909306 ) ) ;
#7301=CARTESIAN_POINT ( 'NONE',  ( 47.75598903798131545, 95.36109484030878036, 32.59926919370181508 ) ) ;
#7308=CARTESIAN_POINT ( 'NONE',  ( 26.67903320394502131, 150.0857490671680807, 9.287084330314211655 ) ) ;
#7311=DIRECTION ( 'NONE',  ( 0.7066505893342458489, 0.7066505893340067068, 0.03591502732094190020 ) ) ;
#7313=CARTESIAN_POINT ( 'NONE',  ( 9.656473946750173454, 127.6128973189080398, 2.339233609801092406 ) ) ;
#7315=CARTESIAN_POINT ( 'NONE',  ( 17.20459894546975832, 108.5405110446994001, 1.704077971530460811 ) ) ;
#7323=CARTESIAN_POINT ( 'NONE',  ( 15.39564893635072806, 140.1373336744895255, -4.208549045858890558 ) ) ;
#7334=CARTESIAN_POINT ( 'NONE',  ( 33.56091001181424360, 87.00402361476987778, -6.351118090676544981 ) ) ;
#7336=DIRECTION ( 'NONE',  ( 0.000000000000000000, 0.000000000000000000, -1.000000000000000000 ) ) ;
#7341=CARTESIAN_POINT ( 'NONE',  ( 48.12388674207330297, 92.25590008057444891, 8.208355790051324874 ) ) ;
#7356=CARTESIAN_POINT ( 'NONE',  ( 52.07920593110389262, 93.11959619657488929, 13.05671643426689776 ) ) ;
#7362=CARTESIAN_POINT ( 'NONE',  ( 75.85495621331871519, 129.5603373922052697, -8.732165470513974626 ) ) ;
#7364=CARTESIAN_POINT ( 'NONE',  ( 54.67410106651116308, 94.23276814491528341, 6.942135068398441078 ) ) ;
#7374=CARTESIAN_POINT ( 'NONE',  ( 73.74613032677598312, 134.8023270448005064, -0.9181577650121128809 ) ) ;
#7376=CARTESIAN_POINT ( 'NONE',  ( 75.40436159597490473, 130.9804297329818326, 12.22031048084446248 ) ) ;
#7383=CARTESIAN_POINT ( 'NONE',  ( 52.46025766099742071, 152.8098426157893925, 11.14871012209260748 ) ) ;
#7391=CARTESIAN_POINT ( 'NONE',  ( 32.24825037804825456, 146.0601464669000791, 9.485560667832931614 ) ) ;
#7401=CARTESIAN_POINT ( 'NONE',  ( 63.17392202723403472, 139.5086487405075673, -1.196242060499778992 ) ) ;
#7406=CARTESIAN_POINT ( 'NONE',  ( 44.62452158104316879, 94.95733355596098590, 29.46674713776154775 ) ) ;
#7414=CARTESIAN_POINT ( 'NONE',  ( 23.80922038702690102, 91.46939207759763235, 0.001460074241615882690 ) ) ;
#7421=CARTESIAN_POINT ( 'NONE',  ( 26.10333545525518062, 97.33820528946348816, 8.132564544556878161 ) ) ;
#7428=CARTESIAN_POINT ( 'NONE',  ( 76.81974253126139729, 125.2811442093199616, -1.589308178208348910 ) ) ;
#7437=CARTESIAN_POINT ( 'NONE',  ( 15.39564893635072806, 140.1373336744895255, -4.208549045858890558 ) ) ;
#7443=CARTESIAN_POINT ( 'NONE',  ( 60.64192606672164487, 149.1585417170215067, -15.56126092485307488 ) ) ;
#7459=CARTESIAN_POINT ( 'NONE',  ( 15.34898554898258460, 114.0222161449793248, 7.937823431466153323 ) ) ;
#7466=CARTESIAN_POINT ( 'NONE',  ( 39.42188022582085694, 153.9507182763122159, -10.27990332573616961 ) ) ;
#7467=CARTESIAN_POINT ( 'NONE',  ( 62.17156016504299032, 99.21662021101468554, 6.584824431686855384 ) ) ;
#7470=EDGE_CURVE ( 'NONE', #11596, #10804, #14929, .T. ) ;
#7481=CARTESIAN_POINT ( 'NONE',  ( 67.48508721674359379, 143.7297851702464015, -1.275552590249036777 ) ) ;
#7489=CARTESIAN_POINT ( 'NONE',  ( 8.867590775667826719, 116.4845415224344833, 7.977433149383395872 ) ) ;
#7496=DIRECTION ( 'NONE',  ( 0.9387810623359077455, 0.3426822732243072211, 0.03548206049944095664 ) ) ;
#7497=CARTESIAN_POINT ( 'NONE',  ( 62.38482844916680392, 99.30468409114129713, 12.58043553469319953 ) ) ;
#7508=CARTESIAN_POINT ( 'NONE',  ( 20.50804704269433998, 103.0453634090187762, -11.55335571609641399 ) ) ;
#7521=CARTESIAN_POINT ( 'NONE',  ( 30.01547214559559507, 151.6658481390280144, 9.406004577920295873 ) ) ;
#7525=EDGE_LOOP ( 'NONE', ( #19852, #1795, #4826, #9641 ) ) ;
#7527=CARTESIAN_POINT ( 'NONE',  ( 57.86150831142030171, 95.93494642397840266, -0.2007220744356660869 ) ) ;
#7534=CARTESIAN_POINT ( 'NONE',  ( 77.24268685965694203, 120.2105100216710696, 12.57728155048203433 ) ) ;
#7538=DIRECTION ( 'NONE',  ( 0.000000000000000000, 0.000000000000000000, 1.000000000000000000 ) ) ;
#7546=CARTESIAN_POINT ( 'NONE',  ( 20.75180444880664510, 93.89949152720284076, -5.875022464008872625 ) ) ;
#7552=CARTESIAN_POINT ( 'NONE',  ( 23.54274795406405474, 91.84646939011692268, -11.98975411606233976 ) ) ;
#7570=CARTESIAN_POINT ( 'NONE',  ( 32.24825037804825456, 146.0601464669000791, 9.485560667832931614 ) ) ;
#7577=CARTESIAN_POINT ( 'NONE',  ( 9.021810916323596885, 123.9851095102452945, 2.220310480865780534 ) ) ;
#7578=CARTESIAN_POINT ( 'NONE',  ( 58.43892221570314405, 143.5117748958429047, 4.561220828673259398 ) ) ;
#7589=CARTESIAN_POINT ( 'NONE',  ( 48.37701604703377001, 153.6359454806530778, -1.989754116034292197 ) ) ;
#7592=CARTESIAN_POINT ( 'NONE',  ( 23.42018083028975184, 147.9700754799198705, 17.16443675223517573 ) ) ;
#7598=CARTESIAN_POINT ( 'NONE',  ( 15.20278999188385960, 140.0102622722330636, 1.787054806504753346 ) ) ;
#7603=CARTESIAN_POINT ( 'NONE',  ( 15.94687047784549172, 111.7036002239776451, 14.84254118869207417 ) ) ;
#7615=CARTESIAN_POINT ( 'NONE',  ( 58.57598713290192904, 143.3259681031794059, -1.434385245616870197 ) ) ;
#7618=CARTESIAN_POINT ( 'NONE',  ( 48.01123829699398726, 144.4020089423098341, 33.87806037135994330 ) ) ;
#7625=CARTESIAN_POINT ( 'NONE',  ( 28.88048086162541850, 151.0887240815949895, -10.63664014359656385 ) ) ;
#7630=CARTESIAN_POINT ( 'NONE',  ( 71.48324150724619130, 139.0594858779678873, 3.930207297951037848 ) ) ;
#7639=CARTESIAN_POINT ( 'NONE',  ( 15.18239976710701100, 124.4615124019231018, 16.34704286353642999 ) ) ;
#7650=CARTESIAN_POINT ( 'NONE',  ( 24.41145734808947054, 148.6458414325078081, 10.19629000755267434 ) ) ;
#7651=CARTESIAN_POINT ( 'NONE',  ( 39.35878039893513858, 95.17507832528838208, 37.62897400776943613 ) ) ;
#7661=CARTESIAN_POINT ( 'NONE',  ( 18.86674891209846905, 143.9013856721611546, -11.04182128657428485 ) ) ;
#7685=CARTESIAN_POINT ( 'NONE',  ( 17.21810733192966936, 108.3100148859214329, 7.699684045823485867 ) ) ;
#7692=CARTESIAN_POINT ( 'NONE',  ( 77.19215121279506775, 118.0176990621192203, -1.351406188750652992 ) ) ;
#7693=CARTESIAN_POINT ( 'NONE',  ( 15.53781593631592983, 113.9137188375014347, -11.07707013084618097 ) ) ;
#7702=CARTESIAN_POINT ( 'NONE',  ( 72.81290617574171620, 103.2231620977376281, 0.1530188383368442095 ) ) ;
#7709=CARTESIAN_POINT ( 'NONE',  ( 47.52490801233957995, 85.89149910694642642, 6.191896081848653921 ) ) ;
#7713=ADVANCED_FACE ( 'NONE', ( #19590 ), #4064, .T. ) ;
#7715=CARTESIAN_POINT ( 'NONE',  ( 68.93731127356984700, 108.6095829621005180, 19.12825547442421126 ) ) ;
#7716=( NAMED_UNIT ( * ) SI_UNIT ( $, .STERADIAN. ) SOLID_ANGLE_UNIT ( ) );
#7725=CARTESIAN_POINT ( 'NONE',  ( 46.34060549886174840, 91.98545359010019240, -5.720099531362743406 ) ) ;
#7734=CARTESIAN_POINT ( 'NONE',  ( 32.98198692859195802, 152.6383102900375093, -3.493975233523312962 ) ) ;
#7740=CARTESIAN_POINT ( 'NONE',  ( 52.27439898384277939, 152.9467924839493946, 17.14431721725165758 ) ) ;
#7749=CARTESIAN_POINT ( 'NONE',  ( 70.51576897149806200, 126.1317638695992116, 12.41827883020830470 ) ) ;
#7756=CARTESIAN_POINT ( 'NONE',  ( 42.68022887774371554, 94.90707761860559799, 39.21067981925356349 ) ) ;
#7765=CARTESIAN_POINT ( 'NONE',  ( 63.55746018358933469, 147.2895578332197033, -9.446739241148069510 ) ) ;
#7766=DIRECTION ( 'NONE',  ( 0.000000000000000000, 0.000000000000000000, 1.000000000000000000 ) ) ;
#7786=CARTESIAN_POINT ( 'NONE',  ( 46.46425003030392986, 147.9761360841216344, 3.056716434341200106 ) ) ;
#7792=CARTESIAN_POINT ( 'NONE',  ( 36.55618291757107841, 153.5264344809625641, -3.375052104409746789 ) ) ;
#7793=CARTESIAN_POINT ( 'NONE',  ( 46.87248680087107999, 147.7605717807558676, -8.934501345478663481 ) ) ;
#7794=CARTESIAN_POINT ( 'NONE',  ( 71.86557814238962294, 101.4853659568252766, -7.779689512009451136 ) ) ;
#7802=CARTESIAN_POINT ( 'NONE',  ( 11.23391594879739941, 132.3357020601377769, 10.49983985543964415 ) ) ;
#7805=CARTESIAN_POINT ( 'NONE',  ( 53.04203944364535772, 87.17698241397053494, 14.00585298808814194 ) ) ;
#7807=SHAPE_REPRESENTATION_RELATIONSHIP ( 'NONE' , 'NONE' ,  #14632, #13479 ) ;
#7811=CARTESIAN_POINT ( 'NONE',  ( 15.82680954991375621, 98.96776360684994245, 0.3584833779906905771 ) ) ;
#7818=CARTESIAN_POINT ( 'NONE',  ( 59.59119729515064279, 96.99641097138604096, 19.72329267725583080 ) ) ;
#7831=CARTESIAN_POINT ( 'NONE',  ( 70.81223827124823345, 124.1306694702586100, -7.505929917039384058 ) ) ;
#7839=CARTESIAN_POINT ( 'NONE',  ( 8.779377865064803999, 119.6051361893432130, -4.922546661887801100 ) ) ;
#7847=CARTESIAN_POINT ( 'NONE',  ( 14.94030450088465400, 100.1727563578744196, 14.40630071170483362 ) ) ;
#7853=CARTESIAN_POINT ( 'NONE',  ( 20.72232308940363765, 137.1362251821529696, 16.90007324815861267 ) ) ;
#7861=CARTESIAN_POINT ( 'NONE',  ( 66.24914683137549787, 94.76885710642066840, 6.506024766557033878 ) ) ;
#7871=CARTESIAN_POINT ( 'NONE',  ( 75.80354157443048280, 110.0810758630161672, 5.910575721798123183 ) ) ;
#7894=CARTESIAN_POINT ( 'NONE',  ( 24.78883071187807730, 141.3519591882296709, -10.86778418981948846 ) ) ;
#7900=CARTESIAN_POINT ( 'NONE',  ( 47.30009524607925897, 85.94413156685014599, 0.1962900075584997628 ) ) ;
#7901=CARTESIAN_POINT ( 'NONE',  ( 66.22715431465987024, 135.7747266163150073, -15.00590082692269078 ) ) ;
#7919=CARTESIAN_POINT ( 'NONE',  ( 71.22865828484523831, 100.3801644121689094, 12.26314743512348926 ) ) ;
#7924=CARTESIAN_POINT ( 'NONE',  ( 71.19430100617981338, 118.9508470517051535, -8.295922056425867552 ) ) ;
#7929=ORIENTED_EDGE ( 'NONE', *, *, #17003, .F. ) ;
#7935=CARTESIAN_POINT ( 'NONE',  ( 15.79683473163509966, 126.9851207307152521, 3.446356185820485418 ) ) ;
#7943=CARTESIAN_POINT ( 'NONE',  ( 39.42188022582085694, 153.9507182763122159, -10.27990332573616961 ) ) ;
#7953=CARTESIAN_POINT ( 'NONE',  ( 65.15795615308765321, 146.1170287843621054, 17.62046751038700165 ) ) ;
#7956=CARTESIAN_POINT ( 'NONE',  ( 51.37827275082728562, 86.79484443300951568, -12.94217320967262275 ) ) ;
#7964=CARTESIAN_POINT ( 'NONE',  ( 37.00104444766353851, 92.35499785847434850, 7.656504971210453370 ) ) ;
#7966=CARTESIAN_POINT ( 'NONE',  ( 75.40436159597490473, 130.9804297329818326, 12.22031048084446248 ) ) ;
#7971=CARTESIAN_POINT ( 'NONE',  ( 42.35458290462738518, 144.9005011087681396, 39.17808643222355869 ) ) ;
#7977=CARTESIAN_POINT ( 'NONE',  ( 76.92284642892752800, 124.5854180935290714, 5.434424407683230207 ) ) ;
#8004=CARTESIAN_POINT ( 'NONE',  ( 30.88693878601983300, 94.35661743609990992, 20.91413290821214588 ) ) ;
#8010=CARTESIAN_POINT ( 'NONE',  ( 30.24639091383375700, 151.6717570033048048, 3.410403464249057492 ) ) ;
#8012=CARTESIAN_POINT ( 'NONE',  ( 14.85320491933239317, 121.4429315054255909, 16.22795414098078126 ) ) ;
#8029=CARTESIAN_POINT ( 'NONE',  ( 11.40453246296876877, 106.5480838228176452, 14.64419766361223552 ) ) ;
#8035=CARTESIAN_POINT ( 'NONE',  ( 50.58784882905466418, 147.1537178454131549, 17.22345644918840790 ) ) ;
#8046=CARTESIAN_POINT ( 'NONE',  ( 53.81137604271221164, 145.8702381773545653, 5.351212940250758443 ) ) ;
#8055=CARTESIAN_POINT ( 'NONE',  ( 8.927628897234525240, 116.7075971571176751, 1.981832035706394546 ) ) ;
#8061=CARTESIAN_POINT ( 'NONE',  ( 32.32016755483360271, 87.30015788337030358, 13.69171886368053492 ) ) ;
#8065=EDGE_CURVE ( 'NONE', #13715, #460, #9299, .T. ) ;
#8066=CARTESIAN_POINT ( 'NONE',  ( 66.55041322599720388, 95.16028120083096553, -6.513516925475251185 ) ) ;
#8069=CARTESIAN_POINT ( 'NONE',  ( 30.72731853479779929, 94.52359049060457608, 14.91853181686295038 ) ) ;
#8075=CARTESIAN_POINT ( 'NONE',  ( 47.24326884731692644, 147.7868190896643341, 4.084992211255583427 ) ) ;
#8086=CARTESIAN_POINT ( 'NONE',  ( 24.41145734808947054, 148.6458414325078081, 10.19629000755267434 ) ) ;
#8108=CARTESIAN_POINT ( 'NONE',  ( 64.05606230151549596, 101.0139342820504993, 19.48556066606253978 ) ) ;
#8114=CARTESIAN_POINT ( 'NONE',  ( 23.42018083028975184, 147.9700754799198705, 17.16443675223517573 ) ) ;
#8117=CARTESIAN_POINT ( 'NONE',  ( 64.45983652262509622, 101.7220219035630748, -6.553643814208265361 ) ) ;
#8130=AXIS2_PLACEMENT_3D ( 'NONE', #16964, #17071, #16751 ) ;
#8134=CARTESIAN_POINT ( 'NONE',  ( 65.15795615308765321, 146.1170287843621054, 17.62046751038700165 ) ) ;
#8139=CARTESIAN_POINT ( 'NONE',  ( 31.13415902118537559, 151.9291573665896635, 4.438733124005141306 ) ) ;
#8141=CARTESIAN_POINT ( 'NONE',  ( 32.78705717043479240, 146.2756902729748560, 16.50925200294354056 ) ) ;
#8152=CARTESIAN_POINT ( 'NONE',  ( 25.52315018325464635, 97.88680518890443238, 9.160641959101482712 ) ) ;
#8163=CARTESIAN_POINT ( 'NONE',  ( 40.90832812944997698, 154.0758954209757121, 3.767805038447253452 ) ) ;
#8171=CARTESIAN_POINT ( 'NONE',  ( 34.18339000214019308, 153.0669919960894845, 16.54886172077450368 ) ) ;
#8174=CARTESIAN_POINT ( 'NONE',  ( 23.40005864183818218, 147.8691531402271835, -9.846981161663094895 ) ) ;
#8183=CARTESIAN_POINT ( 'NONE',  ( 43.01140435219951996, 70.71049967264875136, 29.21067981925357060 ) ) ;
#8187=CARTESIAN_POINT ( 'NONE',  ( 69.49396330798431620, 129.5978393632817927, 5.275421687385184910 ) ) ;
#8198=CARTESIAN_POINT ( 'NONE',  ( 75.16956835342354282, 131.6452004531123805, 5.196376467030073165 ) ) ;
#8204=CARTESIAN_POINT ( 'NONE',  ( 36.55618291757107841, 153.5264344809625641, -3.375052104409746789 ) ) ;
#8205=ORIENTED_EDGE ( 'NONE', *, *, #10963, .F. ) ;
#8213=CARTESIAN_POINT ( 'NONE',  ( 41.83190538388809188, 154.0406478741334126, 4.796127949319595629 ) ) ;
#8222=CARTESIAN_POINT ( 'NONE',  ( 20.52669235689029037, 137.0142703344444897, 22.89568392956547882 ) ) ;
#8228=CARTESIAN_POINT ( 'NONE',  ( 65.27013532398795803, 145.9152199903044504, 11.62486143609835310 ) ) ;
#8230=CARTESIAN_POINT ( 'NONE',  ( 15.11514590861459162, 123.4468881749472615, -3.696500957071167104 ) ) ;
#8247=CARTESIAN_POINT ( 'NONE',  ( 63.06653971011325410, 92.06373373134326243, 19.64449301269484849 ) ) ;
#8251=CARTESIAN_POINT ( 'NONE',  ( 52.81156257015842925, 87.19036605886009283, 8.010245892729333406 ) ) ;
#8252=CARTESIAN_POINT ( 'NONE',  ( 15.53003795322992353, 126.2325256570730687, 2.418278830334454899 ) ) ;
#8264=CARTESIAN_POINT ( 'NONE',  ( 69.89089498905519804, 111.6491328518190613, -0.005813817042542732995 ) ) ;
#8275=CARTESIAN_POINT ( 'NONE',  ( 14.88286428391304561, 100.3963227437532595, 8.410691821786379307 ) ) ;
#8282=CARTESIAN_POINT ( 'NONE',  ( 15.77498628565902727, 140.7233915340666499, 22.81684008552556975 ) ) ;
#8285=CARTESIAN_POINT ( 'NONE',  ( 8.987667018801221985, 116.9306527918008527, -4.013769077970609445 ) ) ;
#8291=CARTESIAN_POINT ( 'NONE',  ( 33.01799438418878907, 146.2770090272405810, 10.51364782838779099 ) ) ;
#8304=CARTESIAN_POINT ( 'NONE',  ( 35.69068542950036260, 86.46542255174357194, 7.577194441455407770 ) ) ;
#8315=CARTESIAN_POINT ( 'NONE',  ( 22.17150742865759483, 138.9041494244890771, -4.010207742755246052 ) ) ;
#8320=CARTESIAN_POINT ( 'NONE',  ( 52.81156257015842925, 87.19036605886009283, 8.010245892729333406 ) ) ;
#8330=CARTESIAN_POINT ( 'NONE',  ( 25.76509531087978289, 97.49384569152056201, 21.15186415193267067 ) ) ;
#8337=CARTESIAN_POINT ( 'NONE',  ( 21.63557314705429846, 101.6375443364048152, 2.375099401820868206 ) ) ;
#8355=CARTESIAN_POINT ( 'NONE',  ( 53.94306145151312393, 87.38125778962682944, 12.97772928308168616 ) ) ;
#8361=CARTESIAN_POINT ( 'NONE',  ( 45.50561661668613311, 153.9697812235645245, 4.915054502968218664 ) ) ;
#8362=CARTESIAN_POINT ( 'NONE',  ( 31.84750084766683287, 94.01163676417708359, 0.8705387173494113506 ) ) ;
#8368=VERTEX_POINT ( 'NONE', #11515 ) ;
#8374=CARTESIAN_POINT ( 'NONE',  ( 16.71508173162657229, 129.8698440624217483, 3.565528294796503683 ) ) ;
#8385=CARTESIAN_POINT ( 'NONE',  ( 63.41425016244589585, 92.41789933959738335, 6.624947895572852019 ) ) ;
#8392=CARTESIAN_POINT ( 'NONE',  ( 68.00896726847550156, 133.1338957242411709, 4.128172222816925085 ) ) ;
#8394=FILL_AREA_STYLE_COLOUR ( '', #17614 ) ;
#8405=CARTESIAN_POINT ( 'NONE',  ( 41.25620118372704326, 148.0523446076144580, 3.846850258842608117 ) ) ;
#8417=CARTESIAN_POINT ( 'NONE',  ( 15.97061701817242785, 140.8453463817331794, 16.82122940411608170 ) ) ;
#8419=ORIENTED_EDGE ( 'NONE', *, *, #5300, .T. ) ;
#8425=CARTESIAN_POINT ( 'NONE',  ( 20.75180444880664510, 93.89949152720284076, -5.875022464008872625 ) ) ;
#8427=CARTESIAN_POINT ( 'NONE',  ( 14.81332417359726783, 119.6334487847019403, -4.843746996953559147 ) ) ;
#8433=CARTESIAN_POINT ( 'NONE',  ( 70.43474449472395804, 99.54920534645194152, 7.295875980836476593 ) ) ;
#8447=CARTESIAN_POINT ( 'NONE',  ( 14.94677925004173957, 122.6663546818147381, -4.724578312614759135 ) ) ;
#8452=CARTESIAN_POINT ( 'NONE',  ( 43.01140435219951996, 119.9070776186055838, -19.99999999999997868 ) ) ;
#8454=CARTESIAN_POINT ( 'NONE',  ( 30.18028515090226449, 151.2280014487717779, 17.43780275515692679 ) ) ;
#8456=CARTESIAN_POINT ( 'NONE',  ( 24.14732448757077776, 99.05405632904258084, -4.767757741039170938 ) ) ;
#8471=CARTESIAN_POINT ( 'NONE',  ( 65.22477088018504787, 102.4029861919955948, -1.586113490162427864 ) ) ;
#8478=CARTESIAN_POINT ( 'NONE',  ( 14.34121205894687456, 138.4663445754194697, 3.724531598165178092 ) ) ;
#8479=CARTESIAN_POINT ( 'NONE',  ( 16.33471683235446292, 110.7640000046674089, -5.200637885961103102 ) ) ;
#8483=CARTESIAN_POINT ( 'NONE',  ( 43.01140435219951996, 119.9070776186055838, 50.00000000000002842 ) ) ;
#8489=CARTESIAN_POINT ( 'NONE',  ( 19.07518309319397432, 143.9976739860571229, -17.03742665657317801 ) ) ;
#8497=CARTESIAN_POINT ( 'NONE',  ( 51.78234217841457365, 152.9971814535558963, 4.124977536042813142 ) ) ;
#8504=CARTESIAN_POINT ( 'NONE',  ( 69.60802376816022274, 110.2920722108499518, -1.943010761821444943 ) ) ;
#8510=DIRECTION ( 'NONE',  ( 0.9387810623359078566, 0.3426822732243069436, 0.03548206049944095664 ) ) ;
#8517=CARTESIAN_POINT ( 'NONE',  ( 26.92635752117756098, 142.9018661569831750, -16.76761354414967542 ) ) ;
#8523=CARTESIAN_POINT ( 'NONE',  ( 39.96017580440467043, 144.7216711109867049, 30.23627618186983312 ) ) ;
#8529=CARTESIAN_POINT ( 'NONE',  ( 55.35048440753327981, 87.88826800209452017, -1.070088050731120344 ) ) ;
#8536=CARTESIAN_POINT ( 'NONE',  ( 9.021810916323596885, 123.9851095102452945, 2.220310480865780534 ) ) ;
#8543=CARTESIAN_POINT ( 'NONE',  ( 38.34086628137072239, 86.07498427433979771, 8.486398261126511855 ) ) ;
#8554=CARTESIAN_POINT ( 'NONE',  ( 50.11350838007777497, 92.61696660072725251, -6.867350599827054758 ) ) ;
#8560=CARTESIAN_POINT ( 'NONE',  ( 21.90415124324598750, 92.95514585177724598, 15.07745334355238676 ) ) ;
#8561=CARTESIAN_POINT ( 'NONE',  ( 70.72621728061167801, 115.1542034346632875, -7.148670959876664455 ) ) ;
#8571=CYLINDRICAL_SURFACE ( 'NONE', #21034, 24.99999999999998934 ) ;
#8576=CARTESIAN_POINT ( 'NONE',  ( 16.32863300717066579, 110.5331391746388761, 0.7949662885976053195 ) ) ;
#8579=CARTESIAN_POINT ( 'NONE',  ( 77.15557362092413030, 120.6950048976143250, -0.4420599252208967100 ) ) ;
#8581=CARTESIAN_POINT ( 'NONE',  ( 24.25535704844963547, 98.85002770340597067, 1.227849354118501601 ) ) ;
#8590=CARTESIAN_POINT ( 'NONE',  ( 76.07019559177007295, 111.3280993686123281, -14.13269547130637704 ) ) ;
#8599=CARTESIAN_POINT ( 'NONE',  ( 26.66797635711824199, 149.9459070286683868, 17.30505193804556185 ) ) ;
#8606=CARTESIAN_POINT ( 'NONE',  ( 70.95506224315714405, 115.5552942049593668, 4.842541188697900623 ) ) ;
#8619=CARTESIAN_POINT ( 'NONE',  ( 29.48178659935447854, 144.5857871963822845, 17.33364154221121467 ) ) ;
#8627=CARTESIAN_POINT ( 'NONE',  ( 38.17209587424806472, 144.4343147008670485, 32.91136586774996431 ) ) ;
#8632=CARTESIAN_POINT ( 'NONE',  ( 9.231363607564425422, 125.4582397780895633, 16.26765482522027639 ) ) ;
#8638=CARTESIAN_POINT ( 'NONE',  ( 42.92180000979148957, 85.67454126555050209, 7.339147150375312734 ) ) ;
#8639=EDGE_LOOP ( 'NONE', ( #8419, #6145 ) ) ;
#8640=CARTESIAN_POINT ( 'NONE',  ( 71.19430100617981338, 118.9508470517051535, -8.295922056425867552 ) ) ;
#8647=CARTESIAN_POINT ( 'NONE',  ( 30.24639091383375700, 151.6717570033048048, 3.410403464249057492 ) ) ;
#8657=CARTESIAN_POINT ( 'NONE',  ( 59.92122946415073415, 142.4742691614619332, -9.367183195626855863 ) ) ;
#8665=CARTESIAN_POINT ( 'NONE',  ( 68.96269327682742301, 142.1111764150114993, -15.20387477620461425 ) ) ;
#8675=DIRECTION ( 'NONE',  ( -1.000000000000000000, 0.000000000000000000, 0.000000000000000000 ) ) ;
#8681=CARTESIAN_POINT ( 'NONE',  ( 35.43645570112151688, 92.65990651318493576, -0.2767073223962682738 ) ) ;
#8685=CARTESIAN_POINT ( 'NONE',  ( 23.67598417054553295, 91.65793073385727041, -5.994147020910363999 ) ) ;
#8686=CARTESIAN_POINT ( 'NONE',  ( 57.86150831142030171, 95.93494642397840266, -0.2007220744356660869 ) ) ;
#8700=CARTESIAN_POINT ( 'NONE',  ( 71.19781441516849441, 139.1947734567256703, -15.08494495145127878 ) ) ;
#8711=CARTESIAN_POINT ( 'NONE',  ( 11.08170843061617816, 132.1625483722078513, 16.49545033792581350 ) ) ;
#8716=CARTESIAN_POINT ( 'NONE',  ( 20.64193819951031017, 102.6032774297415102, 0.4378519886423143381 ) ) ;
#8727=CARTESIAN_POINT ( 'NONE',  ( 60.58642193167724344, 97.95666160567475345, -13.33918631239395225 ) ) ;
#8733=CARTESIAN_POINT ( 'NONE',  ( 46.77777258146056738, 95.19132504939746298, 37.51526355657936307 ) ) ;
#8735=CARTESIAN_POINT ( 'NONE',  ( 38.26853956736072604, 144.4533880425008192, 35.82660397859488199 ) ) ;
#8736=AXIS2_PLACEMENT_3D ( 'NONE', #19111, #7538, #5653 ) ;
#8742=CARTESIAN_POINT ( 'NONE',  ( 38.54497605562327323, 85.96704844161884296, 14.48200433579215662 ) ) ;
#8748=CARTESIAN_POINT ( 'NONE',  ( 10.16827731527805767, 110.2528774685086574, 8.767718578943870966 ) ) ;
#8750=CARTESIAN_POINT ( 'NONE',  ( 17.24633477965345918, 131.3686459745448758, -4.367463884209165315 ) ) ;
#8757=CARTESIAN_POINT ( 'NONE',  ( 54.54805624998882507, 152.1374805055981199, -2.779977617235711129 ) ) ;
#8766=CARTESIAN_POINT ( 'NONE',  ( 62.66823040046688931, 140.1266048904901993, -2.224326160187301227 ) ) ;
#8775=CARTESIAN_POINT ( 'NONE',  ( 61.44294336830710535, 141.1433446673695471, 5.708471897238777792 ) ) ;
#8793=CARTESIAN_POINT ( 'NONE',  ( 28.99223550982291897, 144.4690685518502846, 2.342703524990218611 ) ) ;
#8797=ADVANCED_FACE ( 'NONE', ( #2248 ), #10742, .F. ) ;
#8798=CARTESIAN_POINT ( 'NONE',  ( 33.56091001181424360, 87.00402361476987778, -6.351118090676544981 ) ) ;
#8799=CARTESIAN_POINT ( 'NONE',  ( 26.10333545525518062, 97.33820528946348816, 8.132564544556878161 ) ) ;
#8809=CARTESIAN_POINT ( 'NONE',  ( 9.046145050308979307, 123.4917717844193277, -10.79923121120670437 ) ) ;
#8820=CARTESIAN_POINT ( 'NONE',  ( 12.61881386508366809, 104.1535352963828984, 15.55354899318430739 ) ) ;
#8825=CARTESIAN_POINT ( 'NONE',  ( 60.05828665636081354, 97.34093765924853869, 12.69960079420514809 ) ) ;
#8826=ADVANCED_FACE ( 'NONE', ( #14463 ), #10855, .T. ) ;
#8839=CARTESIAN_POINT ( 'NONE',  ( 25.64412274706724304, 97.69032544021251852, 15.15625305551708202 ) ) ;
#8841=CARTESIAN_POINT ( 'NONE',  ( 45.51311879618403822, 144.7820145757526404, 29.87844397536261098 ) ) ;
#8852=CARTESIAN_POINT ( 'NONE',  ( 42.88582110127141789, 154.2205544383733695, -4.165101255777401867 ) ) ;
#8853=ORIENTED_EDGE ( 'NONE', *, *, #11847, .T. ) ;
#8857=CARTESIAN_POINT ( 'NONE',  ( 35.69068542950036260, 86.46542255174357194, 7.577194441455407770 ) ) ;
#8859=CARTESIAN_POINT ( 'NONE',  ( 64.66009251794113766, 101.8366349233107684, -0.5580327111990067701 ) ) ;
#8865=CARTESIAN_POINT ( 'NONE',  ( 57.78275410301085913, 89.02518083909171764, -0.1607367497116551913 ) ) ;
#8869=CARTESIAN_POINT ( 'NONE',  ( 9.616596702810701558, 112.3753283828585694, -5.161025107254184618 ) ) ;
#8882=CARTESIAN_POINT ( 'NONE',  ( 77.08865571979157494, 122.1823731668103221, -14.48986716664726870 ) ) ;
#8902=CARTESIAN_POINT ( 'NONE',  ( 71.28213884770818254, 119.1643779896719764, -2.300315981272657240 ) ) ;
#8907=CARTESIAN_POINT ( 'NONE',  ( 53.88337135589062399, 152.3674195137575964, -9.803719146365084569 ) ) ;
#8908=CARTESIAN_POINT ( 'NONE',  ( 59.83664469576316236, 97.27638873328486113, 6.703993115985443119 ) ) ;
#8924=CARTESIAN_POINT ( 'NONE',  ( 62.84376099716368458, 92.00366499689042143, 13.64888190966157566 ) ) ;
#8930=CARTESIAN_POINT ( 'NONE',  ( 24.55476856798156859, 141.3345980244743885, 9.128255474432329208 ) ) ;
#8941=CARTESIAN_POINT ( 'NONE',  ( 67.15412698936957270, 134.4792784496449087, 12.06138812558265805 ) ) ;
#8954=CARTESIAN_POINT ( 'NONE',  ( 15.20278999188385960, 140.0102622722330636, 1.787054806504753346 ) ) ;
#8959=CARTESIAN_POINT ( 'NONE',  ( 71.03835150376274044, 100.2492380157770526, 6.267546321443639989 ) ) ;
#8961=CARTESIAN_POINT ( 'NONE',  ( 15.38454125381035098, 114.2504036285165654, 1.942219256913226388 ) ) ;
#8971=CARTESIAN_POINT ( 'NONE',  ( 36.55618291757107841, 153.5264344809625641, -3.375052104409746789 ) ) ;
#8981=CARTESIAN_POINT ( 'NONE',  ( 77.15313604554262383, 122.4041478163663612, -8.494263314424808087 ) ) ;
#8988=CARTESIAN_POINT ( 'NONE',  ( 63.64508858465791974, 100.8029030738736225, 7.494358438614500351 ) ) ;
#9006=CARTESIAN_POINT ( 'NONE',  ( 60.05828665636081354, 97.34093765924853869, 12.69960079420514809 ) ) ;
#9012=CARTESIAN_POINT ( 'NONE',  ( 13.69124840528610321, 102.2378096837820181, -5.517995706778950016 ) ) ;
#9013=CARTESIAN_POINT ( 'NONE',  ( 45.98873144221455789, 91.86516812052268222, 7.299390993452533394 ) ) ;
#9023=CARTESIAN_POINT ( 'NONE',  ( 69.07271358049158039, 97.83220508185358710, -6.632443479277712051 ) ) ;
#9032=CARTESIAN_POINT ( 'NONE',  ( 41.61242760320212852, 154.1118385459532760, 10.79173905232880237 ) ) ;
#9040=CARTESIAN_POINT ( 'NONE',  ( 70.99289463508769416, 124.0080672713295087, 11.50917073501047483 ) ) ;
#9050=CARTESIAN_POINT ( 'NONE',  ( 29.95680074317227692, 144.8134228754239530, -2.624813489111333720 ) ) ;
#9064=CARTESIAN_POINT ( 'NONE',  ( 10.28555834757860055, 130.2242880576791890, 1.430031502841225821 ) ) ;
#9071=CARTESIAN_POINT ( 'NONE',  ( 31.84750084766683287, 94.01163676417708359, 0.8705387173494113506 ) ) ;
#9072=EDGE_LOOP ( 'NONE', ( #21703, #10833, #2007, #925 ) ) ;
#9078=CARTESIAN_POINT ( 'NONE',  ( 71.53613896966024299, 138.8348963267899592, -2.065403804986401859 ) ) ;
#9092=CARTESIAN_POINT ( 'NONE',  ( 71.14040157825178312, 139.4183699182763974, -9.089337262093875935 ) ) ;
#9099=CARTESIAN_POINT ( 'NONE',  ( 36.14055301128134801, 147.1744539460121075, 4.637215583376333328 ) ) ;
#9119=CARTESIAN_POINT ( 'NONE',  ( 64.86034851325717909, 101.9512479430583625, 5.437578391810254708 ) ) ;
#9124=CARTESIAN_POINT ( 'NONE',  ( 61.61057083318216598, 91.16763906547615193, -7.303593892219363504 ) ) ;
#9125=CARTESIAN_POINT ( 'NONE',  ( 15.96294818963569639, 111.9339314265907745, 8.846935114401974332 ) ) ;
#9135=CARTESIAN_POINT ( 'NONE',  ( 30.47730968207189051, 151.6776658675815384, -2.585197649422186661 ) ) ;
#9137=CARTESIAN_POINT ( 'NONE',  ( 68.29446192123552350, 96.82662215664792882, 13.41040346623746515 ) ) ;
#9143=CARTESIAN_POINT ( 'NONE',  ( 11.68597903420391226, 105.9017562933008918, 7.620467510411443435 ) ) ;
#9151=CARTESIAN_POINT ( 'NONE',  ( 22.18708823908250238, 100.7722391081675255, 7.342430719951936524 ) ) ;
#9156=EDGE_LOOP ( 'NONE', ( #6434, #4606 ) ) ;
#9162=CARTESIAN_POINT ( 'NONE',  ( 15.65696388169908104, 126.4253507882334588, -3.577328847893908925 ) ) ;
#9174=CARTESIAN_POINT ( 'NONE',  ( 13.37233465371036090, 102.6159639102351093, 7.501340520787425525 ) ) ;
#9182=CARTESIAN_POINT ( 'NONE',  ( 40.57367117788501787, 91.81261228707245436, 0.5136478283763052932 ) ) ;
#9189=CARTESIAN_POINT ( 'NONE',  ( 76.40658810299491677, 127.4365358892444959, 12.33923360994393903 ) ) ;
#9191=EDGE_CURVE ( 'NONE', #4997, #18531, #15172, .T. ) ;
#9199=CARTESIAN_POINT ( 'NONE',  ( 9.616596702810701558, 112.3753283828585694, -5.161025107254184618 ) ) ;
#9205=CARTESIAN_POINT ( 'NONE',  ( 9.127117681521182746, 124.1904119534442401, -3.775300622140596030 ) ) ;
#9226=CARTESIAN_POINT ( 'NONE',  ( 14.87688376430095616, 117.0300574687981481, 8.056989239287382532 ) ) ;
#9232=CARTESIAN_POINT ( 'NONE',  ( 76.81974253126139729, 125.2811442093199616, -1.589308178208348910 ) ) ;
#9233=CARTESIAN_POINT ( 'NONE',  ( 55.81398226145393693, 145.0329042473489096, 4.442248136324586483 ) ) ;
#9244=CARTESIAN_POINT ( 'NONE',  ( 63.19260820189420969, 92.35335041358771946, 0.6293402173502762320 ) ) ;
#9248=CARTESIAN_POINT ( 'NONE',  ( 31.20897972572539558, 148.4098837309084900, 17.43780275515693390 ) ) ;
#9251=CARTESIAN_POINT ( 'NONE',  ( 30.25101221841200427, 88.05347211559326581, -0.2365872832861977970 ) ) ;
#9256=CARTESIAN_POINT ( 'NONE',  ( 29.49905557571407044, 144.7517438296894738, 9.366394860000250233 ) ) ;
#9266=CARTESIAN_POINT ( 'NONE',  ( 52.67254683800726411, 146.3150465326280028, -8.696212858991016148 ) ) ;
#9268=CARTESIAN_POINT ( 'NONE',  ( 47.50526184765048754, 144.5001958438514009, 36.42700876960374501 ) ) ;
#9280=CARTESIAN_POINT ( 'NONE',  ( 43.59077634914400079, 154.2158251336064723, 2.858602931426994953 ) ) ;
#9287=CARTESIAN_POINT ( 'NONE',  ( 24.77189431714078083, 141.4131305960171687, 3.132649400142189844 ) ) ;
#9294=CARTESIAN_POINT ( 'NONE',  ( 21.43032318156618388, 146.4805633285969861, 10.07716523980869816 ) ) ;
#9295=CARTESIAN_POINT ( 'NONE',  ( 39.24942077270426211, 95.19152545906743512, 37.50829531803063333 ) ) ;
#9299=CIRCLE ( 'NONE', #17027, 10.00000000000000888 ) ;
#9304=CARTESIAN_POINT ( 'NONE',  ( 64.11693453485118255, 146.8606268255622638, -2.422805558527139080 ) ) ;
#9305=CARTESIAN_POINT ( 'NONE',  ( 43.01140435219951996, 119.9070776186055838, 8.284271247461942878 ) ) ;
#9328=CARTESIAN_POINT ( 'NONE',  ( 68.00896726847550156, 133.1338957242411709, 4.128172222816925085 ) ) ;
#9331=DIRECTION ( 'NONE',  ( 0.000000000000000000, 0.000000000000000000, -1.000000000000000000 ) ) ;
#9333=CARTESIAN_POINT ( 'NONE',  ( 50.92548328124963319, 86.60151408976496157, 0.07716523989554470442 ) ) ;
#9334=CARTESIAN_POINT ( 'NONE',  ( 18.82712405543679779, 105.5606057458561793, -11.43438524559667790 ) ) ;
#9335=CARTESIAN_POINT ( 'NONE',  ( 17.73005198514846725, 142.9879744078657779, -4.089424278207452801 ) ) ;
#9345=CARTESIAN_POINT ( 'NONE',  ( 9.504183449854689769, 113.2927979568517571, -4.132695447411913747 ) ) ;
#9352=CARTESIAN_POINT ( 'NONE',  ( 8.916504151126011024, 123.7798070670463773, 8.215921583872152212 ) ) ;
#9360=CARTESIAN_POINT ( 'NONE',  ( 70.05982654948900290, 127.8813624167294023, -8.653178033719973072 ) ) ;
#9371=CARTESIAN_POINT ( 'NONE',  ( 24.58042389364637259, 98.66975071380154816, -11.79164420265881574 ) ) ;
#9386=ORIENTED_EDGE ( 'NONE', *, *, #4507, .F. ) ;
#9388=CARTESIAN_POINT ( 'NONE',  ( 22.95395889711706872, 147.7494453258605915, 2.144227187454380790 ) ) ;
#9395=CARTESIAN_POINT ( 'NONE',  ( 41.83412315030695794, 148.0818998446914634, 10.87053871734362431 ) ) ;
#9403=CARTESIAN_POINT ( 'NONE',  ( 25.52397925108762067, 90.47728371212039633, 7.934596195134201224 ) ) ;
#9414=CARTESIAN_POINT ( 'NONE',  ( 10.61900875472251649, 108.8314319666055212, -5.279948415675857376 ) ) ;
#9443=CARTESIAN_POINT ( 'NONE',  ( 38.01409278319488294, 147.7425775668531003, 9.723292677533123651 ) ) ;
#9450=CARTESIAN_POINT ( 'NONE',  ( 76.66991938639012005, 113.6622739410785670, 5.791450954060403333 ) ) ;
#9451=CARTESIAN_POINT ( 'NONE',  ( 15.80414578680225723, 112.4924633436790344, 15.87081086175909306 ) ) ;
#9459=CARTESIAN_POINT ( 'NONE',  ( 14.43535904578935103, 101.2031681353820574, 9.438814132600386486 ) ) ;
#9463=CARTESIAN_POINT ( 'NONE',  ( 21.43032318156618388, 146.4805633285969861, 10.07716523980869816 ) ) ;
#9469=CARTESIAN_POINT ( 'NONE',  ( 61.24245875951225315, 90.83725678726602837, 5.715745788549559059 ) ) ;
#9475=CARTESIAN_POINT ( 'NONE',  ( 40.03295031927941494, 147.9482203214073479, -10.20071078494585670 ) ) ;
#9486=CARTESIAN_POINT ( 'NONE',  ( 32.21091799184858218, 93.94358800413606048, -12.14875741943239085 ) ) ;
#9489=CARTESIAN_POINT ( 'NONE',  ( 43.34257982665531728, 144.9070776186055696, 39.21067981925357060 ) ) ;
#9495=CARTESIAN_POINT ( 'NONE',  ( 77.22348061889915982, 118.7203125366680752, -8.375138532479306619 ) ) ;
#9503=CARTESIAN_POINT ( 'NONE',  ( 75.94266982333172677, 110.2653427511449422, 11.90618179609112026 ) ) ;
#9518=CARTESIAN_POINT ( 'NONE',  ( 35.69068542950036260, 86.46542255174357194, 7.577194441455407770 ) ) ;
#9519=CARTESIAN_POINT ( 'NONE',  ( 38.52064617801426749, 95.31338828682366682, 31.98784611697848135 ) ) ;
#9528=CARTESIAN_POINT ( 'NONE',  ( 36.38086904327614235, 86.32171732562966326, 0.5532606071062302622 ) ) ;
#9549=CARTESIAN_POINT ( 'NONE',  ( 15.53544334784188585, 126.6048195653137469, 15.43757839183889224 ) ) ;
#9555=CARTESIAN_POINT ( 'NONE',  ( 20.88913110926514705, 146.0313881486468119, 3.053432864643822686 ) ) ;
#9556=CARTESIAN_POINT ( 'NONE',  ( 26.87902611899987448, 142.9395564687116007, -9.767670631928341507 ) ) ;
#9565=CARTESIAN_POINT ( 'NONE',  ( 68.08897506277223499, 96.72110655255949041, 7.414802352519190620 ) ) ;
#9573=CARTESIAN_POINT ( 'NONE',  ( 22.95395889711706872, 147.7494453258605915, 2.144227187454380790 ) ) ;
#9581=CARTESIAN_POINT ( 'NONE',  ( 69.69253243162556544, 129.2828754355126648, 18.29472124897268159 ) ) ;
#9589=AXIS2_PLACEMENT_3D ( 'NONE', #20294, #8510, #9943 ) ;
#9593=CARTESIAN_POINT ( 'NONE',  ( 61.95829188091916961, 99.12855633088805973, 0.5892133286805102399 ) ) ;
#9602=CARTESIAN_POINT ( 'NONE',  ( 15.39564893635072806, 140.1373336744895255, -4.208549045858890558 ) ) ;
#9607=EDGE_LOOP ( 'NONE', ( #14010, #10159, #17768, #19089 ) ) ;
#9611=CARTESIAN_POINT ( 'NONE',  ( 30.67228459367742133, 151.9265198579663263, 16.42994147312239051 ) ) ;
#9614=CARTESIAN_POINT ( 'NONE',  ( 73.15003751907750029, 103.8404476760371864, -6.870911935119222491 ) ) ;
#9616=ORIENTED_EDGE ( 'NONE', *, *, #11847, .F. ) ;
#9622=CARTESIAN_POINT ( 'NONE',  ( 15.53003795322992353, 126.2325256570730687, 2.418278830334454899 ) ) ;
#9624=CARTESIAN_POINT ( 'NONE',  ( 30.90322180743143576, 151.9278386122780375, 10.43433729856376502 ) ) ;
#9625=CARTESIAN_POINT ( 'NONE',  ( 38.26843650118725293, 95.36078014034055172, 32.59446367923827381 ) ) ;
#9628=CARTESIAN_POINT ( 'NONE',  ( 42.68014329765944126, 144.9070776186055696, 39.21067981925356349 ) ) ;
#9634=CARTESIAN_POINT ( 'NONE',  ( 9.822352152143091431, 128.2981216602131553, 9.363167623699879982 ) ) ;
#9641=ORIENTED_EDGE ( 'NONE', *, *, #18588, .F. ) ;
#9642=ORIENTED_EDGE ( 'NONE', *, *, #333, .T. ) ;
#9658=CARTESIAN_POINT ( 'NONE',  ( 44.65913741311992879, 148.1402468479653578, 16.98531508000710843 ) ) ;
#9663=CARTESIAN_POINT ( 'NONE',  ( 43.01140435219951996, 70.71049967264875136, 34.21067981925357060 ) ) ;
#9664=CARTESIAN_POINT ( 'NONE',  ( 48.17517050666977241, 153.7480039124125994, 4.005852979123367241 ) ) ;
#9666=CARTESIAN_POINT ( 'NONE',  ( 66.60919851020621252, 104.6140855887898624, -13.69650096386476079 ) ) ;
#9685=CARTESIAN_POINT ( 'NONE',  ( 20.67200536010596323, 145.9528555770810385, 9.049038938933962939 ) ) ;
#9691=CARTESIAN_POINT ( 'NONE',  ( 39.55749537675153960, 91.83829536962669238, 20.55682687220188143 ) ) ;
#9700=CARTESIAN_POINT ( 'NONE',  ( 33.35040633798650589, 93.49848361726675705, 8.803757759246650494 ) ) ;
#9710=CARTESIAN_POINT ( 'NONE',  ( 36.38086904327614235, 86.32171732562966326, 0.5532606071062302622 ) ) ;
#9717=CARTESIAN_POINT ( 'NONE',  ( 75.17075062522994244, 131.8760474256973509, 11.19198414525841301 ) ) ;
#9720=CARTESIAN_POINT ( 'NONE',  ( 54.88857506304572809, 87.88569651147935247, -13.06129575545291210 ) ) ;
#9725=CARTESIAN_POINT ( 'NONE',  ( 59.36841858216658352, 96.93634223693318575, 13.72768157422830981 ) ) ;
#9732=CARTESIAN_POINT ( 'NONE',  ( 29.12819380265916180, 95.36133955912156068, 0.9897074016940036190 ) ) ;
#9735=CARTESIAN_POINT ( 'NONE',  ( 38.01157040740503845, 95.41214629490136190, 33.87806037135995751 ) ) ;
#9744=CARTESIAN_POINT ( 'NONE',  ( 61.76154402333882132, 148.5480768402654803, 4.482004293238171400 ) ) ;
#9768=CARTESIAN_POINT ( 'NONE',  ( 23.10700517764660589, 139.6571016847272233, -10.96257334342637435 ) ) ;
#9775=CARTESIAN_POINT ( 'NONE',  ( 38.54497605562327323, 85.96704844161884296, 14.48200433579215662 ) ) ;
#9777=CARTESIAN_POINT ( 'NONE',  ( 32.23767430054685690, 145.5917660130465379, 17.43780275515692679 ) ) ;
#9795=CARTESIAN_POINT ( 'NONE',  ( 47.97332496630577481, 153.8600623441721211, 10.00146007428102379 ) ) ;
#9800=CARTESIAN_POINT ( 'NONE',  ( 53.48172298457406271, 87.39834721931525507, 0.9865115032505324955 ) ) ;
#9802=CARTESIAN_POINT ( 'NONE',  ( 65.96530660583994177, 103.3855952397044007, 19.36639486037446289 ) ) ;
#9811=CARTESIAN_POINT ( 'NONE',  ( 19.47480796662762970, 104.5210170170265229, 9.517959287447121497 ) ) ;
#9819=CARTESIAN_POINT ( 'NONE',  ( 26.90790578767411390, 150.1165885900122987, 3.291480155758420345 ) ) ;
#9826=CARTESIAN_POINT ( 'NONE',  ( 24.18607167610233333, 148.5957190367184353, 16.19189608183989648 ) ) ;
#9828=CARTESIAN_POINT ( 'NONE',  ( 58.10477600886401461, 150.5438954262070581, -8.656458923931941385 ) ) ;
#9838=CARTESIAN_POINT ( 'NONE',  ( 40.57367117788501787, 91.81261228707245436, 0.5136478283763052932 ) ) ;
#9840=CARTESIAN_POINT ( 'NONE',  ( 9.231363607564425422, 125.4582397780895633, 16.26765482522027639 ) ) ;
#9849=CARTESIAN_POINT ( 'NONE',  ( 29.43094928344231320, 88.48265962617873015, 0.7917390523231137012 ) ) ;
#9855=CARTESIAN_POINT ( 'NONE',  ( 44.41273964558330789, 85.70220254879866673, -6.708519844216274564 ) ) ;
#9864=PRODUCT_DEFINITION_FORMATION_WITH_SPECIFIED_SOURCE ( 'ANY', '', #19990, .NOT_KNOWN. ) ;
#9873=CARTESIAN_POINT ( 'NONE',  ( 26.61521700243209310, 142.9206948758876194, 23.22567064538713666 ) ) ;
#9880=CARTESIAN_POINT ( 'NONE',  ( 31.47436479266152531, 87.67613096727390598, 14.72005176623422606 ) ) ;
#9882=CARTESIAN_POINT ( 'NONE',  ( 38.46765184765857981, 147.6574975633170936, -2.267929528491105629 ) ) ;
#9899=CARTESIAN_POINT ( 'NONE',  ( 75.73800832010900308, 109.5907576069244698, 18.92991194937467014 ) ) ;
#9904=CARTESIAN_POINT ( 'NONE',  ( 68.08897506277223499, 96.72110655255949041, 7.414802352519190620 ) ) ;
#9905=CARTESIAN_POINT ( 'NONE',  ( 55.29376081731632553, 145.2908078538121401, -2.581636314160848489 ) ) ;
#9915=CARTESIAN_POINT ( 'NONE',  ( 70.62278752756289180, 114.5844828164671441, -0.1247842873985126749 ) ) ;
#9928=CARTESIAN_POINT ( 'NONE',  ( 25.52397925108762067, 90.47728371212039633, 7.934596195134201224 ) ) ;
#9936=CARTESIAN_POINT ( 'NONE',  ( 76.97284262070103011, 124.8108046395131225, 11.43003150283799663 ) ) ;
#9938=CARTESIAN_POINT ( 'NONE',  ( 69.07271358049158039, 97.83220508185358710, -6.632443479277712051 ) ) ;
#9943=DIRECTION ( 'NONE',  ( -0.3428981916074324565, 0.9393725726208703719, 0.000000000000000000 ) ) ;
#9949=CARTESIAN_POINT ( 'NONE',  ( 19.23080508249268661, 135.0620028898917440, 9.799277925644819476 ) ) ;
#9962=CARTESIAN_POINT ( 'NONE',  ( 73.72238702602700755, 135.0318370961144296, 5.077453337991364002 ) ) ;
#9968=CARTESIAN_POINT ( 'NONE',  ( 76.04618105687035268, 128.8835079444423286, -1.708432735116285350 ) ) ;
#9970=CARTESIAN_POINT ( 'NONE',  ( 20.25093610150840107, 136.5556286039603435, -4.129180435126924564 ) ) ;
#9975=CARTESIAN_POINT ( 'NONE',  ( 60.49690154327523572, 149.3382625450468311, -9.565656633516235630 ) ) ;
#9986=CARTESIAN_POINT ( 'NONE',  ( 71.28758990370504023, 120.3962046462169440, 18.65202787790538608 ) ) ;
#9993=CARTESIAN_POINT ( 'NONE',  ( 41.61242760320212852, 154.1118385459532760, 10.79173905232880237 ) ) ;
#9994=CARTESIAN_POINT ( 'NONE',  ( 71.07673676950255981, 118.1590465568689581, -7.267641430287227422 ) ) ;
#10009=CARTESIAN_POINT ( 'NONE',  ( 76.97284262070103011, 124.8108046395131225, 11.43003150283799663 ) ) ;
#10014=CARTESIAN_POINT ( 'NONE',  ( 75.39856087065255963, 130.7497677300756607, 6.224699377836747871 ) ) ;
#10015=CARTESIAN_POINT ( 'NONE',  ( 27.10205971394288582, 96.62443569844734270, -5.915007788698968483 ) ) ;
#10026=CARTESIAN_POINT ( 'NONE',  ( 69.49278103613195867, 129.3669923906968222, -0.7201859908431552659 ) ) ;
#10029=CYLINDRICAL_SURFACE ( 'NONE', #5518, 24.99999999999998934 ) ;
#10038=CARTESIAN_POINT ( 'NONE',  ( 8.869018199820361659, 117.4101421016551967, 9.005765870029716069 ) ) ;
#10046=CARTESIAN_POINT ( 'NONE',  ( 39.80927132972225024, 148.0054509460111660, -4.205104553811644941 ) ) ;
#10056=CARTESIAN_POINT ( 'NONE',  ( 15.66613903973849986, 126.7949701480144711, 9.441967288829692606 ) ) ;
#10063=CARTESIAN_POINT ( 'NONE',  ( 38.45534370351731468, 144.4885014985149496, 32.14446507322553970 ) ) ;
#10068=CARTESIAN_POINT ( 'NONE',  ( 72.33162239183086228, 137.5781058455011703, 11.98183203572534872 ) ) ;
#10074=CARTESIAN_POINT ( 'NONE',  ( 53.88337135589062399, 152.3674195137575964, -9.803719146365084569 ) ) ;
#10081=CARTESIAN_POINT ( 'NONE',  ( 75.10802748102119608, 108.0013139708956800, -8.018167963582932600 ) ) ;
#10092=CARTESIAN_POINT ( 'NONE',  ( 34.72595348466361287, 146.8618156516888291, -3.415175568290148345 ) ) ;
#10097=PLANE ( 'NONE',  #4848 ) ;
#10098=CARTESIAN_POINT ( 'NONE',  ( 30.90322180743143576, 151.9278386122780375, 10.43433729856376502 ) ) ;
#10100=CARTESIAN_POINT ( 'NONE',  ( 18.53657114080759527, 106.0614633106838909, -4.410498573173142312 ) ) ;
#10101=AXIS2_PLACEMENT_3D ( 'NONE', #9305, #7336, #14245 ) ;
#10117=CARTESIAN_POINT ( 'NONE',  ( 76.78854507624612324, 113.8604396784633508, 11.78705480642107517 ) ) ;
#10124=CARTESIAN_POINT ( 'NONE',  ( 75.16838608161717161, 131.4143534805274101, -0.7992312111982662337 ) ) ;
#10125=CARTESIAN_POINT ( 'NONE',  ( 14.93692188586762803, 117.2531131035273546, 2.061388125607503952 ) ) ;
#10137=CARTESIAN_POINT ( 'NONE',  ( 17.93535261252752022, 143.0936276526352913, -10.08503035249478685 ) ) ;
#10146=CARTESIAN_POINT ( 'NONE',  ( 66.89036333300305159, 144.4373801540182569, -2.303882249869787291 ) ) ;
#10155=CARTESIAN_POINT ( 'NONE',  ( 41.36127970224624306, 91.67401929561202678, -0.5144393322287174053 ) ) ;
#10159=ORIENTED_EDGE ( 'NONE', *, *, #9191, .F. ) ;
#10168=CARTESIAN_POINT ( 'NONE',  ( 71.07552608251525328, 117.1481954606975791, 12.77539325861266484 ) ) ;
#10171=CARTESIAN_POINT ( 'NONE',  ( 9.976645104453018220, 110.9295780357170571, 15.79146183154218619 ) ) ;
#10180=CARTESIAN_POINT ( 'NONE',  ( 49.46632042442519861, 86.28835692931116341, 14.12497754236212977 ) ) ;
#10187=CARTESIAN_POINT ( 'NONE',  ( 75.16956835342354282, 131.6452004531123805, 5.196376467030073165 ) ) ;
#10190=( LENGTH_UNIT ( ) NAMED_UNIT ( * ) SI_UNIT ( .MILLI., .METRE. ) );
#10195=CARTESIAN_POINT ( 'NONE',  ( 49.23863765798637360, 86.32632880410874066, 8.129368652084252744 ) ) ;
#10205=CARTESIAN_POINT ( 'NONE',  ( 17.24633477965345918, 131.3686459745448758, -4.367463884209165315 ) ) ;
#10212=CARTESIAN_POINT ( 'NONE',  ( 14.15704070161504369, 138.3271338521546454, 9.720138693322796897 ) ) ;
#10214=CARTESIAN_POINT ( 'NONE',  ( 70.81223827124823345, 124.1306694702586100, -7.505929917039384058 ) ) ;
#10223=FACE_OUTER_BOUND ( 'NONE', #13770, .T. ) ;
#10228=CARTESIAN_POINT ( 'NONE',  ( 23.20524185134216921, 147.9029287973646660, 23.16022673208204807 ) ) ;
#10233=CARTESIAN_POINT ( 'NONE',  ( 69.90255027150604406, 140.9627200460241454, -1.156626220813373518 ) ) ;
#10234=CARTESIAN_POINT ( 'NONE',  ( 60.38095089740433252, 142.1228462996803046, -2.343495028824083004 ) ) ;
#10246=CARTESIAN_POINT ( 'NONE',  ( 10.62509257988331335, 109.0622927966340967, -11.27555259023744405 ) ) ;
#10255=CARTESIAN_POINT ( 'NONE',  ( 75.40436159597490473, 130.9804297329818326, 12.22031048084446248 ) ) ;
#10261=CARTESIAN_POINT ( 'NONE',  ( 66.11232864078046134, 136.2219195394164899, -3.014685448219384334 ) ) ;
#10272=CARTESIAN_POINT ( 'NONE',  ( 70.22564533444385404, 112.8265553529472953, -14.05338489394683243 ) ) ;
#10276=DIRECTION ( 'NONE',  ( -0.000000000000000000, 1.000000000000000000, -0.000000000000000000 ) ) ;
#10284=CARTESIAN_POINT ( 'NONE',  ( 77.24268685965694203, 120.2105100216710696, 12.57728155048203433 ) ) ;
#10292=CARTESIAN_POINT ( 'NONE',  ( 57.14511974427749408, 88.72838517433189054, 6.862995836283489304 ) ) ;
#10295=CARTESIAN_POINT ( 'NONE',  ( 43.06284635655732274, 148.1064719378950088, -10.08176808973812655 ) ) ;
#10301=CARTESIAN_POINT ( 'NONE',  ( 8.927628897234525240, 116.7075971571176751, 1.981832035706394546 ) ) ;
#10312=CARTESIAN_POINT ( 'NONE',  ( 70.05982654948900290, 127.8813624167294023, -8.653178033719973072 ) ) ;
#10320=CARTESIAN_POINT ( 'NONE',  ( 69.49278103613195867, 129.3669923906968222, -0.7201859908431552659 ) ) ;
#10336=CARTESIAN_POINT ( 'NONE',  ( 32.55111017628423298, 93.63144033427927582, -0.1575420629755377999 ) ) ;
#10340=CARTESIAN_POINT ( 'NONE',  ( 43.10205244623161036, 154.1398065127551149, -10.16071067355346358 ) ) ;
#10341=CARTESIAN_POINT ( 'NONE',  ( 67.98812442775457043, 106.8157236907426153, -0.7957547315468347371 ) ) ;
#10352=CARTESIAN_POINT ( 'NONE',  ( 58.10477600886401461, 150.5438954262070581, -8.656458923931941385 ) ) ;
#10363=CARTESIAN_POINT ( 'NONE',  ( 55.94180145820917716, 151.6039095241057453, 11.26783467880839140 ) ) ;
#10369=CARTESIAN_POINT ( 'NONE',  ( 57.25245068215419053, 144.3413351293631877, -3.490753295080526453 ) ) ;
#10382=CARTESIAN_POINT ( 'NONE',  ( 15.16534570839878349, 115.4582699162533288, 15.98979919289822149 ) ) ;
#10390=CARTESIAN_POINT ( 'NONE',  ( 38.67287161060778544, 144.5284399170337792, 36.71770137080346785 ) ) ;
#10395=CARTESIAN_POINT ( 'NONE',  ( 77.07719282571002850, 116.5297446719512209, 12.69640610750513865 ) ) ;
#10401=CARTESIAN_POINT ( 'NONE',  ( 51.78234217841457365, 152.9971814535558963, 4.124977536042813142 ) ) ;
#10403=CARTESIAN_POINT ( 'NONE',  ( 50.11350838007777497, 92.61696660072725251, -6.867350599827054758 ) ) ;
#10409=CARTESIAN_POINT ( 'NONE',  ( 40.02721236285810136, 85.80382532021769748, 0.4343372985580923329 ) ) ;
#10417=CARTESIAN_POINT ( 'NONE',  ( 20.25093610150840107, 136.5556286039603435, -4.129180435126924564 ) ) ;
#10426=CARTESIAN_POINT ( 'NONE',  ( 67.19681472375953035, 134.2522627023263908, 6.065787011912938453 ) ) ;
#10431=APPLICATION_CONTEXT ( 'automotive_design' ) ;
#10446=CARTESIAN_POINT ( 'NONE',  ( 66.97710950389229367, 104.8926460354658587, -1.705278757464820938 ) ) ;
#10450=CARTESIAN_POINT ( 'NONE',  ( 71.14040157825178312, 139.4183699182763974, -9.089337262093875935 ) ) ;
#10452=CARTESIAN_POINT ( 'NONE',  ( 15.66613903973849986, 126.7949701480144711, 9.441967288829692606 ) ) ;
#10463=CARTESIAN_POINT ( 'NONE',  ( 54.72474920843421131, 151.9887481548900325, -8.775581469602226292 ) ) ;
#10474=CARTESIAN_POINT ( 'NONE',  ( 49.46632042442519861, 86.28835692931116341, 14.12497754236212977 ) ) ;
#10479=CARTESIAN_POINT ( 'NONE',  ( 50.34320592624661828, 92.59351467088818310, -0.8717445255428065698 ) ) ;
#10489=CARTESIAN_POINT ( 'NONE',  ( 69.68673170630326297, 129.0522134326295145, 12.29911014595921692 ) ) ;
#10492=CARTESIAN_POINT ( 'NONE',  ( 44.31111858724877095, 144.8753732970614863, 29.37128083581765381 ) ) ;
#10494=CARTESIAN_POINT ( 'NONE',  ( 43.33818195800462547, 94.90707761860556957, 29.21067981925357060 ) ) ;
#10503=CARTESIAN_POINT ( 'NONE',  ( 60.35187701982888342, 149.5179833730722407, -3.570052342179399485 ) ) ;
#10509=CARTESIAN_POINT ( 'NONE',  ( 66.76198117565915879, 95.25264312590786631, -0.5179092472497510702 ) ) ;
#10511=CARTESIAN_POINT ( 'NONE',  ( 14.93692188586762803, 117.2531131035273546, 2.061388125607503952 ) ) ;
#10520=CARTESIAN_POINT ( 'NONE',  ( 8.779377865064803999, 119.6051361893432130, -4.922546661887801100 ) ) ;
#10524=CARTESIAN_POINT ( 'NONE',  ( 15.75986397150585816, 99.18880659646561071, -5.637120474378671808 ) ) ;
#10535=CARTESIAN_POINT ( 'NONE',  ( 74.63589561985200760, 132.8035080205385157, -14.84689682711585768 ) ) ;
#10551=CARTESIAN_POINT ( 'NONE',  ( 28.23826046203858908, 88.93502212982269839, 20.83457506318435648 ) ) ;
#10556=CARTESIAN_POINT ( 'NONE',  ( 8.922311181598237440, 122.0085103898528018, 10.15299703236346573 ) ) ;
#10558=CARTESIAN_POINT ( 'NONE',  ( 19.85370653151704090, 103.8158566922722486, 8.489678972899794118 ) ) ;
#10568=CARTESIAN_POINT ( 'NONE',  ( 17.98086284713512129, 132.6641746743869135, 10.68742175872072409 ) ) ;
#10583=CARTESIAN_POINT ( 'NONE',  ( 18.61283035262889385, 105.6058852300018032, 7.580709131559767222 ) ) ;
#10593=CARTESIAN_POINT ( 'NONE',  ( 56.80456144658707274, 95.31062238922963559, 13.84685026556700116 ) ) ;
#10607=CARTESIAN_POINT ( 'NONE',  ( 11.87357267856223864, 134.3244722033052767, 8.572888645784400907 ) ) ;
#10612=CARTESIAN_POINT ( 'NONE',  ( 11.67247064774405452, 106.1322524520788875, 1.624861436118421043 ) ) ;
#10614=CARTESIAN_POINT ( 'NONE',  ( 54.67410106651116308, 94.23276814491528341, 6.942135068398441078 ) ) ;
#10622=CARTESIAN_POINT ( 'NONE',  ( 33.56091001181424360, 87.00402361476987778, -6.351118090676544981 ) ) ;
#10628=UNCERTAINTY_MEASURE_WITH_UNIT (LENGTH_MEASURE( 1.000000000000000082E-05 ), #12225, 'distance_accuracy_value', 'NONE');
#10636=CARTESIAN_POINT ( 'NONE',  ( 43.10205244623161036, 154.1398065127551149, -10.16071067355346358 ) ) ;
#10642=CARTESIAN_POINT ( 'NONE',  ( 50.95956618318000864, 146.8798181090472212, 5.232242258870305918 ) ) ;
#10661=CARTESIAN_POINT ( 'NONE',  ( 42.84661501159713026, 148.1872198635363134, -4.086158671962061284 ) ) ;
#10666=CARTESIAN_POINT ( 'NONE',  ( 26.28921445626723852, 149.7786157371718616, -3.732453678475698311 ) ) ;
#10667=CARTESIAN_POINT ( 'NONE',  ( 42.37836782381873491, 91.71465960395167372, 14.44224817795539373 ) ) ;
#10675=CARTESIAN_POINT ( 'NONE',  ( 8.886384673113061794, 121.3059481585812733, 3.129088064915290346 ) ) ;
#10677=CARTESIAN_POINT ( 'NONE',  ( 59.73150498404358899, 90.03452709159309109, 13.76780503130795097 ) ) ;
#10683=CARTESIAN_POINT ( 'NONE',  ( 21.90415124324598750, 92.95514585177724598, 15.07745334355238676 ) ) ;
#10690=CARTESIAN_POINT ( 'NONE',  ( 19.91114674846567922, 103.5922903064164302, 14.48528786281536895 ) ) ;
#10702=CARTESIAN_POINT ( 'NONE',  ( 19.10471955674299238, 134.7123306330852870, -3.220215631267630219 ) ) ;
#10709=CARTESIAN_POINT ( 'NONE',  ( 45.22896085152458312, 95.00377825571473522, 29.71740844387221969 ) ) ;
#10716=CARTESIAN_POINT ( 'NONE',  ( 9.433072040199128594, 112.8364229897773470, 7.858512901693939234 ) ) ;
#10723=CARTESIAN_POINT ( 'NONE',  ( 24.25535704844963547, 98.85002770340597067, 1.227849354118501601 ) ) ;
#10732=CARTESIAN_POINT ( 'NONE',  ( 12.03843011909301453, 134.4860913190374561, 2.577281550626734141 ) ) ;
#10741=FACE_OUTER_BOUND ( 'NONE', #11032, .T. ) ;
#10742=CYLINDRICAL_SURFACE ( 'NONE', #4441, 4.999999999999997335 ) ;
#10747=CARTESIAN_POINT ( 'NONE',  ( 33.35040633798650589, 93.49848361726675705, 8.803757759246650494 ) ) ;
#10765=CARTESIAN_POINT ( 'NONE',  ( 70.23874406963963679, 127.5525917602273012, 4.366313592093098883 ) ) ;
#10769=ORIENTED_EDGE ( 'NONE', *, *, #17566, .T. ) ;
#10771=CARTESIAN_POINT ( 'NONE',  ( 49.23863765798637360, 86.32632880410874066, 8.129368652084252744 ) ) ;
#10772=CARTESIAN_POINT ( 'NONE',  ( 71.19791805076843616, 120.7596060772701776, 5.632536115698772328 ) ) ;
#10782=CARTESIAN_POINT ( 'NONE',  ( 18.41688673663920284, 143.6040338654656523, -3.061295755333778512 ) ) ;
#10784=CARTESIAN_POINT ( 'NONE',  ( 9.203281625063985061, 114.5318647093721864, 15.91056058043385413 ) ) ;
#10790=CARTESIAN_POINT ( 'NONE',  ( 40.23585178891228509, 85.70481357498144348, 6.429941473113898631 ) ) ;
#10798=CARTESIAN_POINT ( 'NONE',  ( 15.34898554898258460, 114.0222161449793248, 7.937823431466153323 ) ) ;
#10804=VERTEX_POINT ( 'NONE', #16680 ) ;
#10810=CARTESIAN_POINT ( 'NONE',  ( 18.82712405543679779, 105.5606057458561793, -11.43438524559667790 ) ) ;
#10815=CARTESIAN_POINT ( 'NONE',  ( 32.23767430054768823, 145.5917660130458842, 17.43780275515694456 ) ) ;
#10826=CARTESIAN_POINT ( 'NONE',  ( 17.52475135776945336, 142.8823211630961794, 1.906181796079885027 ) ) ;
#10833=ORIENTED_EDGE ( 'NONE', *, *, #5579, .T. ) ;
#10834=CARTESIAN_POINT ( 'NONE',  ( 18.92353847440636727, 134.5693106245527702, 2.775393258647981920 ) ) ;
#10843=CARTESIAN_POINT ( 'NONE',  ( 14.88286428391304561, 100.3963227437532595, 8.410691821786379307 ) ) ;
#10847=CARTESIAN_POINT ( 'NONE',  ( 43.01140435219951286, 94.90707761860558378, 39.21067981925356349 ) ) ;
#10848=APPLICATION_CONTEXT ( 'automotive_design' ) ;
#10854=CARTESIAN_POINT ( 'NONE',  ( 66.76198117565915879, 95.25264312590786631, -0.5179092472497510702 ) ) ;
#10855=CYLINDRICAL_SURFACE ( 'NONE', #10101, 10.00000000000000888 ) ;
#10860=CARTESIAN_POINT ( 'NONE',  ( 65.57965399412842089, 103.1314161556117028, 7.375186511277089352 ) ) ;
#10877=CARTESIAN_POINT ( 'NONE',  ( 24.36338960932843634, 98.64599907776933208, 7.223456449276175029 ) ) ;
#10883=CARTESIAN_POINT ( 'NONE',  ( 12.03843011909301453, 134.4860913190374561, 2.577281550626734141 ) ) ;
#10884=CARTESIAN_POINT ( 'NONE',  ( 58.92189266798492042, 143.1894642327317513, 11.58510527907202992 ) ) ;
#10893=CARTESIAN_POINT ( 'NONE',  ( 25.37887452999470028, 90.65668055682171200, 1.938985092122112563 ) ) ;
#10895=CARTESIAN_POINT ( 'NONE',  ( 14.48810111090402941, 100.9784058478479523, 15.43442115621699529 ) ) ;
#10900=CARTESIAN_POINT ( 'NONE',  ( 73.37616494982036386, 135.8902282719419077, 4.049127002338204662 ) ) ;
#10907=CARTESIAN_POINT ( 'NONE',  ( 62.98455118117477980, 139.9299249275418617, 10.79496628861178387 ) ) ;
#10916=CARTESIAN_POINT ( 'NONE',  ( 15.42009695863806229, 114.4785911120537634, -4.053384917639696994 ) ) ;
#10923=CARTESIAN_POINT ( 'NONE',  ( 20.75180444880664510, 93.89949152720284076, -5.875022464008872625 ) ) ;
#10928=CARTESIAN_POINT ( 'NONE',  ( 18.00183652574411397, 143.4013020786237860, 8.929911949387623338 ) ) ;
#10934=ORIENTED_EDGE ( 'NONE', *, *, #1181, .F. ) ;
#10935=CARTESIAN_POINT ( 'NONE',  ( 38.24087231542673493, 147.7000375650850970, 3.727681574521009900 ) ) ;
#10943=CARTESIAN_POINT ( 'NONE',  ( 53.71239221804358976, 87.38980250447106357, 6.982120393166105998 ) ) ;
#10944=CIRCLE ( 'NONE', #8130, 24.99999999999999289 ) ;
#10953=CARTESIAN_POINT ( 'NONE',  ( 40.73010619540765020, 85.74955863377461185, -6.589596535617429751 ) ) ;
#10963=EDGE_CURVE ( 'NONE', #1853, #13715, #17408, .T. ) ;
#10973=CARTESIAN_POINT ( 'NONE',  ( 58.30185729850432352, 143.6975816885063750, 10.55682690296339032 ) ) ;
#10979=CARTESIAN_POINT ( 'NONE',  ( 9.656473946750173454, 127.6128973189080398, 2.339233609801092406 ) ) ;
#10980=CARTESIAN_POINT ( 'NONE',  ( 49.21618705061847265, 147.3337112213800140, -15.83906960951095577 ) ) ;
#10992=CARTESIAN_POINT ( 'NONE',  ( 57.55288598684787615, 89.00415807515548750, -6.156345639627279986 ) ) ;
#10994=CARTESIAN_POINT ( 'NONE',  ( 52.46025766099742071, 152.8098426157893925, 11.14871012209260748 ) ) ;
#10996=LINE ( 'NONE', #17601, #20589 ) ;
#10999=CARTESIAN_POINT ( 'NONE',  ( 36.32848368193762667, 153.5644447507555981, 2.620555573812929584 ) ) ;
#11005=CARTESIAN_POINT ( 'NONE',  ( 44.65913741311992879, 148.1402468479653578, 16.98531508000710843 ) ) ;
#11015=CARTESIAN_POINT ( 'NONE',  ( 68.06566224877710169, 132.6756899087416457, -7.863043133634088910 ) ) ;
#11017=CARTESIAN_POINT ( 'NONE',  ( 43.01140435219952707, 144.9070776186055696, 39.21067981925356349 ) ) ;
#11022=CARTESIAN_POINT ( 'NONE',  ( 8.944919112598912037, 123.2842988173194385, -4.803623532975393573 ) ) ;
#11028=CARTESIAN_POINT ( 'NONE',  ( 73.49404125747247463, 104.1488224428393039, 5.120290292223307560 ) ) ;
#11032=EDGE_LOOP ( 'NONE', ( #13025, #12274, #17229, #10934 ) ) ;
#11034=CARTESIAN_POINT ( 'NONE',  ( 33.01799438418878907, 146.2770090272405810, 10.51364782838779099 ) ) ;
#11041=CARTESIAN_POINT ( 'NONE',  ( 57.14511974427749408, 88.72838517433189054, 6.862995836283489304 ) ) ;
#11042=CARTESIAN_POINT ( 'NONE',  ( 38.67454084765554256, 95.28543445581169635, 31.70117790783977796 ) ) ;
#11051=CARTESIAN_POINT ( 'NONE',  ( 36.55618291757107841, 153.5264344809625641, -3.375052104409746789 ) ) ;
#11075=CARTESIAN_POINT ( 'NONE',  ( 68.27453032555700929, 132.6178071945132046, 11.15186410612756696 ) ) ;
#11081=EDGE_CURVE ( 'NONE', #8368, #19976, #3705, .T. ) ;
#11082=CARTESIAN_POINT ( 'NONE',  ( 66.24914683137549787, 94.76885710642066840, 6.506024766557033878 ) ) ;
#11083=CARTESIAN_POINT ( 'NONE',  ( 71.10646316465144423, 118.7373161137383732, -14.29152813157908319 ) ) ;
#11084=CARTESIAN_POINT ( 'NONE',  ( 33.56091001181424360, 87.00402361476987778, -6.351118090676544981 ) ) ;
#11095=CARTESIAN_POINT ( 'NONE',  ( 66.03587854725165585, 94.68079322629401418, 0.5104136635535641009 ) ) ;
#11098=CARTESIAN_POINT ( 'NONE',  ( 77.24268685965694203, 120.2105100216710696, 12.57728155048203433 ) ) ;
#11103=CARTESIAN_POINT ( 'NONE',  ( 33.74677389505396263, 86.86730044589080535, -0.3555069876874490942 ) ) ;
#11110=CARTESIAN_POINT ( 'NONE',  ( 20.52669235689029037, 137.0142703344444897, 22.89568392956547882 ) ) ;
#11122=CARTESIAN_POINT ( 'NONE',  ( 47.44511438772692458, 147.6747606579048409, -1.910614883896327054 ) ) ;
#11124=CARTESIAN_POINT ( 'NONE',  ( 46.66402830546390845, 144.6390769119227855, 37.62897400776943613 ) ) ;
#11131=CARTESIAN_POINT ( 'NONE',  ( 13.69124840528610321, 102.2378096837820181, -5.517995706778950016 ) ) ;
#11137=CARTESIAN_POINT ( 'NONE',  ( 77.17837728419731036, 116.7372127726149245, 18.69201499742705153 ) ) ;
#11143=CARTESIAN_POINT ( 'NONE',  ( 51.29519266978688563, 92.95216133272363379, 14.08499220319455780 ) ) ;
#11144=COLOUR_RGB ( '', 0.40784314, 0.44705882, 0.49803922) ;
#11151=CARTESIAN_POINT ( 'NONE',  ( 70.26356658872128946, 140.6255928306487704, 11.86290872716119615 ) ) ;
#11161=CARTESIAN_POINT ( 'NONE',  ( 9.021810916323596885, 123.9851095102452945, 2.220310480865780534 ) ) ;
#11185=CARTESIAN_POINT ( 'NONE',  ( 67.11143925497957241, 134.7062941969633414, 18.05698923925237764 ) ) ;
#11191=ADVANCED_FACE ( 'NONE', ( #4392 ), #12673, .T. ) ;
#11192=CARTESIAN_POINT ( 'NONE',  ( 37.24990543953586553, 153.6521207556136517, 3.648881909465930828 ) ) ;
#11194=CARTESIAN_POINT ( 'NONE',  ( 25.00529828370466490, 141.4305569644042464, -16.86339438981633876 ) ) ;
#11202=CARTESIAN_POINT ( 'NONE',  ( 18.86674891209846905, 143.9013856721611546, -11.04182128657428485 ) ) ;
#11209=CARTESIAN_POINT ( 'NONE',  ( 44.63232748576950115, 85.63068390643836381, -0.7129156696548789585 ) ) ;
#11211=DIRECTION ( 'NONE',  ( -0.3428981916074306802, 0.9393725726208711491, 0.000000000000000000 ) ) ;
#11214=CARTESIAN_POINT ( 'NONE',  ( 65.02675087932300357, 102.2843278501921418, -7.581721168364237151 ) ) ;
#11224=CARTESIAN_POINT ( 'NONE',  ( 14.95244176413730131, 118.0514569880088231, 3.089472225200239563 ) ) ;
#11234=CARTESIAN_POINT ( 'NONE',  ( 76.20123706073158587, 111.5182621349952257, -8.137091297256032973 ) ) ;
#11242=CARTESIAN_POINT ( 'NONE',  ( 31.65106594408818097, 87.52743543124788062, 20.71565594656193454 ) ) ;
#11245=CARTESIAN_POINT ( 'NONE',  ( 64.23777839346797691, 146.6638261710672566, -8.418409733082999225 ) ) ;
#11254=CARTESIAN_POINT ( 'NONE',  ( 10.91571581598819662, 131.8149664739095783, 9.482090752819161139 ) ) ;
#11255=CARTESIAN_POINT ( 'NONE',  ( 40.94616811940298362, 94.99207055061751248, 29.65421901078122602 ) ) ;
#11261=CLOSED_SHELL ( 'NONE', ( #4488, #11359, #8826, #14936, #14195, #11636, #20480, #4593, #8797 ) ) ;
#11266=CARTESIAN_POINT ( 'NONE',  ( 32.14050509837299785, 87.44534670509604268, 7.696117750009315195 ) ) ;
#11273=SURFACE_STYLE_FILL_AREA ( #19661 ) ;
#11291=CARTESIAN_POINT ( 'NONE',  ( 70.00144543033923128, 111.4600545017090241, 19.00928056007509070 ) ) ;
#11296=CARTESIAN_POINT ( 'NONE',  ( 13.33420504782278293, 102.8437529505761603, 1.505736668420971869 ) ) ;
#11297=CARTESIAN_POINT ( 'NONE',  ( 57.54249972904700172, 143.9818934734506115, -15.48196187774845356 ) ) ;
#11314=CARTESIAN_POINT ( 'NONE',  ( 75.94266982333172677, 110.2653427511449422, 11.90618179609112026 ) ) ;
#11320=CARTESIAN_POINT ( 'NONE',  ( 23.10700517764660589, 139.6571016847272233, -10.96257334342637435 ) ) ;
#11332=CARTESIAN_POINT ( 'NONE',  ( 15.97902590142590462, 112.1642626292039324, 2.851329040111875823 ) ) ;
#11342=CARTESIAN_POINT ( 'NONE',  ( 37.24990543953586553, 153.6521207556136517, 3.648881909465930828 ) ) ;
#11349=CARTESIAN_POINT ( 'NONE',  ( 55.77169822954404310, 151.7599422098969910, 17.26344356872107255 ) ) ;
#11353=CARTESIAN_POINT ( 'NONE',  ( 18.41688673663920284, 143.6040338654656523, -3.061295755333778512 ) ) ;
#11357=CARTESIAN_POINT ( 'NONE',  ( 71.20918238807936973, 120.1790618917378879, 12.65642078274776416 ) ) ;
#11359=ADVANCED_FACE ( 'NONE', ( #4724, #13023 ), #10029, .T. ) ;
#11364=CARTESIAN_POINT ( 'NONE',  ( 38.24087231542673493, 147.7000375650850970, 3.727681574521009900 ) ) ;
#11368=CARTESIAN_POINT ( 'NONE',  ( 39.03656800816600736, 95.22440407761430947, 31.15999777443385454 ) ) ;
#11376=CARTESIAN_POINT ( 'NONE',  ( 12.03843011909301453, 134.4860913190374561, 2.577281550626734141 ) ) ;
#11397=CARTESIAN_POINT ( 'NONE',  ( 17.64326796073342862, 132.3496329740814303, 22.67862939001841127 ) ) ;
#11404=CARTESIAN_POINT ( 'NONE',  ( 62.84376099716368458, 92.00366499689042143, 13.64888190966157566 ) ) ;
#11405=CARTESIAN_POINT ( 'NONE',  ( 16.30727314429931241, 128.7156746967485788, -10.48204345529337189 ) ) ;
#11407=ORIENTED_EDGE ( 'NONE', *, *, #17355, .F. ) ;
#11422=CARTESIAN_POINT ( 'NONE',  ( 18.00183652574411397, 143.4013020786237860, 8.929911949387623338 ) ) ;
#11429=CARTESIAN_POINT ( 'NONE',  ( 19.58029209685692962, 104.0714924419353480, 21.50917333468608561 ) ) ;
#11440=CARTESIAN_POINT ( 'NONE',  ( 30.56769828357572294, 94.69056354510921381, 8.922930725513751327 ) ) ;
#11451=CARTESIAN_POINT ( 'NONE',  ( 76.79083979644461522, 114.3551126354810492, -1.232281421064668869 ) ) ;
#11457=CARTESIAN_POINT ( 'NONE',  ( 28.23826046203858908, 88.93502212982269839, 20.83457506318435648 ) ) ;
#11461=CARTESIAN_POINT ( 'NONE',  ( 71.58903643207423784, 138.6103067756119742, -8.061014907923841122 ) ) ;
#11464=CARTESIAN_POINT ( 'NONE',  ( 65.44800906011916197, 136.9904114405718758, 11.94221925691594777 ) ) ;
#11470=CARTESIAN_POINT ( 'NONE',  ( 18.57470074671828542, 105.8336742703428257, 1.585105279193314010 ) ) ;
#11484=CARTESIAN_POINT ( 'NONE',  ( 45.29500579500201951, 154.0643053174194961, 10.91066218119221709 ) ) ;
#11492=CARTESIAN_POINT ( 'NONE',  ( 39.42188022582085694, 153.9507182763122159, -10.27990332573616961 ) ) ;
#11512=CARTESIAN_POINT ( 'NONE',  ( 26.22827968769296092, 97.14409021710402214, 14.12817222279094942 ) ) ;
#11515=CARTESIAN_POINT ( 'NONE',  ( 43.01140435219951996, 144.9070776186055696, 29.21067981925357060 ) ) ;
#11516=EDGE_LOOP ( 'NONE', ( #4042, #4385, #9616, #13366 ) ) ;
#11520=CARTESIAN_POINT ( 'NONE',  ( 32.71008791447857789, 146.0719641954536883, -2.505641559509553140 ) ) ;
#11527=AXIS2_PLACEMENT_3D ( 'NONE', #9663, #18127, #19795 ) ;
#11539=CARTESIAN_POINT ( 'NONE',  ( 76.43728072391715500, 127.6653364257898744, 18.33484128816649772 ) ) ;
#11545=CARTESIAN_POINT ( 'NONE',  ( 72.37431012622080573, 137.3510900982057308, 5.986230922049878167 ) ) ;
#11546=CARTESIAN_POINT ( 'NONE',  ( 29.22050282933603071, 144.5044581412665536, -3.652897588741476742 ) ) ;
#11557=CARTESIAN_POINT ( 'NONE',  ( 14.91610048035210312, 121.0785340954179645, 3.208644154750278865 ) ) ;
#11567=CARTESIAN_POINT ( 'NONE',  ( 76.66991938639012005, 113.6622739410785670, 5.791450954060403333 ) ) ;
#11574=CARTESIAN_POINT ( 'NONE',  ( 45.08439497331802670, 154.1588294112744677, 16.90626985941621641 ) ) ;
#11577=CARTESIAN_POINT ( 'NONE',  ( 47.68298272704948459, 153.7393326413893817, -9.013488496775837078 ) ) ;
#11588=CARTESIAN_POINT ( 'NONE',  ( 18.92353847440636727, 134.5693106245527702, 2.775393258647981920 ) ) ;
#11590=CARTESIAN_POINT ( 'NONE',  ( 18.14018356548558941, 143.3940520581896862, 16.92415443696469879 ) ) ;
#11596=VERTEX_POINT ( 'NONE', #1944 ) ;
#11599=CARTESIAN_POINT ( 'NONE',  ( 76.66991938639012005, 113.6622739410785670, 5.791450954060403333 ) ) ;
#11607=CARTESIAN_POINT ( 'NONE',  ( 71.53613896966024299, 138.8348963267899592, -2.065403804986401859 ) ) ;
#11609=CARTESIAN_POINT ( 'NONE',  ( 69.45715107853048664, 110.1171555912624740, -7.938611875467805667 ) ) ;
#11615=CARTESIAN_POINT ( 'NONE',  ( 31.13415902118537559, 151.9291573665896635, 4.438733124005141306 ) ) ;
#11624=CARTESIAN_POINT ( 'NONE',  ( 50.58784882905466418, 147.1537178454131549, 17.22345644918840790 ) ) ;
#11628=CARTESIAN_POINT ( 'NONE',  ( 26.66797635711824199, 149.9459070286683868, 17.30505193804556185 ) ) ;
#11630=CARTESIAN_POINT ( 'NONE',  ( 67.53959295026429288, 106.1551078129065075, 0.2323293680688409690 ) ) ;
#11636=ADVANCED_FACE ( 'NONE', ( #10223, #5459 ), #8571, .T. ) ;
#11646=CARTESIAN_POINT ( 'NONE',  ( 75.17075062522994244, 131.8760474256973509, 11.19198414525841301 ) ) ;
#11650=CARTESIAN_POINT ( 'NONE',  ( 14.82542406694137860, 100.6198891296320994, 2.415082931867933880 ) ) ;
#11651=CARTESIAN_POINT ( 'NONE',  ( 38.24087231542673493, 147.7000375650850970, 3.727681574521009900 ) ) ;
#11661=CARTESIAN_POINT ( 'NONE',  ( 69.71546013739904879, 111.0973159356150717, 7.018072855358342466 ) ) ;
#11669=AXIS2_PLACEMENT_3D ( 'NONE', #1901, #7311, #14012 ) ;
#11674=CARTESIAN_POINT ( 'NONE',  ( 26.13368487350976110, 90.12329638092472806, 0.9106621812756837686 ) ) ;
#11682=CARTESIAN_POINT ( 'NONE',  ( 37.44377528459369131, 147.6348322250013894, 2.699600794211013621 ) ) ;
#11694=CARTESIAN_POINT ( 'NONE',  ( 65.09246388851926213, 137.4469437283422906, 4.918530982704383270 ) ) ;
#11696=CARTESIAN_POINT ( 'NONE',  ( 26.66797635711824199, 149.9459070286683868, 17.30505193804556185 ) ) ;
#11700=CARTESIAN_POINT ( 'NONE',  ( 38.17211394134016444, 144.4343190729016442, 35.51056251760059723 ) ) ;
#11705=CARTESIAN_POINT ( 'NONE',  ( 20.69791174355615837, 145.8831102580302570, -4.951040100860263138 ) ) ;
#11713=CARTESIAN_POINT ( 'NONE',  ( 18.86674891209848326, 143.9013856721611546, -11.04182128657428485 ) ) ;
#11715=CARTESIAN_POINT ( 'NONE',  ( 29.22050282933603071, 144.5044581412665536, -3.652897588741476742 ) ) ;
#11720=CARTESIAN_POINT ( 'NONE',  ( 77.15313604554262383, 122.4041478163663612, -8.494263314424808087 ) ) ;
#11731=CARTESIAN_POINT ( 'NONE',  ( 67.98812442775457043, 106.8157236907426153, -0.7957547315468347371 ) ) ;
#11737=CARTESIAN_POINT ( 'NONE',  ( 75.59501567365037999, 109.4093883240155378, 12.93430809701916750 ) ) ;
#11739=CARTESIAN_POINT ( 'NONE',  ( 51.61786746416480298, 93.13668562621728597, 1.065498654441493720 ) ) ;
#11745=CARTESIAN_POINT ( 'NONE',  ( 184.5838786899744832, 207.5897843508632263, 23.27362312593913174 ) ) ;
#11756=CARTESIAN_POINT ( 'NONE',  ( 51.59368247783319816, 153.1301807948854616, 10.12058642595840929 ) ) ;
#11761=CARTESIAN_POINT ( 'NONE',  ( 75.45202302719175691, 109.2280190411066059, 6.938704244663667531 ) ) ;
#11763=CARTESIAN_POINT ( 'NONE',  ( 44.18632541912793243, 91.73153706005567187, -6.629209314582290347 ) ) ;
#11776=CARTESIAN_POINT ( 'NONE',  ( 71.58903643207423784, 138.6103067756119742, -8.061014907923841122 ) ) ;
#11786=CARTESIAN_POINT ( 'NONE',  ( 9.656473946750173454, 127.6128973189080398, 2.339233609801092406 ) ) ;
#11794=CARTESIAN_POINT ( 'NONE',  ( 26.48090744323847190, 142.7828511622217889, -4.776412194962503577 ) ) ;
#11805=CARTESIAN_POINT ( 'NONE',  ( 41.83412315030695794, 148.0818998446914634, 10.87053871734362431 ) ) ;
#11814=CARTESIAN_POINT ( 'NONE',  ( 39.70855384287648349, 144.6890526212906991, 30.44250125826515685 ) ) ;
#11819=CARTESIAN_POINT ( 'NONE',  ( 18.65831473100296023, 143.8050973582651579, -5.046215916575388150 ) ) ;
#11825=CARTESIAN_POINT ( 'NONE',  ( 73.72238702602700755, 135.0318370961144296, 5.077453337991364002 ) ) ;
#11828=CARTESIAN_POINT ( 'NONE',  ( 62.66823040046688931, 140.1266048904901993, -2.224326160187301227 ) ) ;
#11835=CARTESIAN_POINT ( 'NONE',  ( 70.33053884415087964, 140.4045759698336724, 5.867304552604015733 ) ) ;
#11845=CARTESIAN_POINT ( 'NONE',  ( 65.02675087932300357, 102.2843278501921418, -7.581721168364237151 ) ) ;
#11847=EDGE_CURVE ( 'NONE', #460, #13715, #5900, .T. ) ;
#11852=CARTESIAN_POINT ( 'NONE',  ( 62.34613790317991544, 148.1570561279473850, 11.50573666851796339 ) ) ;
#11853=CARTESIAN_POINT ( 'NONE',  ( 59.61500273516548276, 97.21183980732109831, 0.7083854377657419210 ) ) ;
#11869=CARTESIAN_POINT ( 'NONE',  ( 8.737656864016759783, 121.5850998216562431, 22.14420391595633220 ) ) ;
#11874=CARTESIAN_POINT ( 'NONE',  ( 75.66441332552922461, 109.8968089748874064, -0.08503035249486777525 ) ) ;
#11875=CARTESIAN_POINT ( 'NONE',  ( 20.57499262110235350, 102.8243204193801432, -5.557751863727047770 ) ) ;
#11887=CARTESIAN_POINT ( 'NONE',  ( 40.51949181395973199, 85.84442682937354618, -12.58519764931165241 ) ) ;
#11896=CARTESIAN_POINT ( 'NONE',  ( 12.43312601512511151, 135.2277911470865490, 16.60371454366222466 ) ) ;
#11903=CARTESIAN_POINT ( 'NONE',  ( 20.05807715703862470, 136.4285572017038248, 1.866423417236719118 ) ) ;
#11915=CARTESIAN_POINT ( 'NONE',  ( 66.22715431465987024, 135.7747266163150073, -15.00590082692269078 ) ) ;
#11920=CARTESIAN_POINT ( 'NONE',  ( 46.98674312866067737, 95.22448645226677399, 31.16068397573690163 ) ) ;
#11927=CARTESIAN_POINT ( 'NONE',  ( 68.29446192123552350, 96.82662215664792882, 13.41040346623746515 ) ) ;
#11933=CARTESIAN_POINT ( 'NONE',  ( 47.30009524607925897, 85.94413156685014599, 0.1962900075584997628 ) ) ;
#11938=CARTESIAN_POINT ( 'NONE',  ( 66.79315400704923888, 104.7533658121278819, -7.700889860664787534 ) ) ;
#11943=CARTESIAN_POINT ( 'NONE',  ( 75.39856087065255963, 130.7497677300756607, 6.224699377836747871 ) ) ;
#11952=CARTESIAN_POINT ( 'NONE',  ( 64.66009251794113766, 101.8366349233107684, -0.5580327111990067701 ) ) ;
#11960=CARTESIAN_POINT ( 'NONE',  ( 29.95680074317227692, 144.8134228754239530, -2.624813489111333720 ) ) ;
#11977=CARTESIAN_POINT ( 'NONE',  ( 69.03752116822961682, 130.9715778530742227, -2.776543650264200025 ) ) ;
#11982=CARTESIAN_POINT ( 'NONE',  ( 35.25059181783574758, 92.79662968204097240, -6.272318425388238694 ) ) ;
#11991=CARTESIAN_POINT ( 'NONE',  ( 69.52170837389681424, 98.37355370181180092, -13.65637406972050272 ) ) ;
#12000=CARTESIAN_POINT ( 'NONE',  ( 42.88582110127141789, 154.2205544383733695, -4.165101255777401867 ) ) ;
#12005=CARTESIAN_POINT ( 'NONE',  ( 55.13406075593908895, 145.4575617026882526, 3.413969760132236964 ) ) ;
#12017=CARTESIAN_POINT ( 'NONE',  ( 66.60919851020621252, 104.6140855887898624, -13.69650096386476079 ) ) ;
#12023=CARTESIAN_POINT ( 'NONE',  ( 38.52630149208098942, 144.5015896161360445, 31.99467674420384355 ) ) ;
#12030=CARTESIAN_POINT ( 'NONE',  ( 9.203281625063985061, 114.5318647093721864, 15.91056058043385413 ) ) ;
#12039=CARTESIAN_POINT ( 'NONE',  ( 25.52397925108762067, 90.47728371212039633, 7.934596195134201224 ) ) ;
#12042=CARTESIAN_POINT ( 'NONE',  ( 41.15066532084431827, 91.76888749123396849, -6.510040445920065366 ) ) ;
#12048=CARTESIAN_POINT ( 'NONE',  ( 13.69124840528610321, 102.2378096837820181, -5.517995706778950016 ) ) ;
#12055=CARTESIAN_POINT ( 'NONE',  ( 66.16974147772015158, 135.9983230778657344, -9.010293137571032673 ) ) ;
#12065=CARTESIAN_POINT ( 'NONE',  ( 29.68407903333335085, 144.6596297928226988, 11.33750686376150085 ) ) ;
#12082=CARTESIAN_POINT ( 'NONE',  ( 61.02373258766779429, 98.10483126312279012, -1.347972122102980119 ) ) ;
#12086=CARTESIAN_POINT ( 'NONE',  ( 9.997522862669264043, 111.1595821513141402, 9.795857695845493041 ) ) ;
#12087=CARTESIAN_POINT ( 'NONE',  ( 59.36841858216658352, 96.93634223693318575, 13.72768157422830981 ) ) ;
#12092=PLANE ( 'NONE',  #18275 ) ;
#12095=CARTESIAN_POINT ( 'NONE',  ( 36.78388215320455856, 153.4884242111695301, -9.370659782632428048 ) ) ;
#12106=CARTESIAN_POINT ( 'NONE',  ( 16.30372524420941716, 141.3216567370616019, 9.839263250375132941 ) ) ;
#12112=CARTESIAN_POINT ( 'NONE',  ( 66.97710950389229367, 104.8926460354658587, -1.705278757464820938 ) ) ;
#12121=CARTESIAN_POINT ( 'NONE',  ( 43.96673757894181023, 91.80305570246190427, -12.62481348914368873 ) ) ;
#12127=CARTESIAN_POINT ( 'NONE',  ( 47.97937126593587465, 95.40557542420955883, 34.86469163422184181 ) ) ;
#12134=CARTESIAN_POINT ( 'NONE',  ( 74.27779736592162863, 105.9683817680885056, 13.05343286460986363 ) ) ;
#12139=CARTESIAN_POINT ( 'NONE',  ( 12.03843011909301453, 134.4860913190374561, 2.577281550626734141 ) ) ;
#12141=CARTESIAN_POINT ( 'NONE',  ( 42.95897134029118547, 91.70801217734280897, 7.418363685804686192 ) ) ;
#12150=CARTESIAN_POINT ( 'NONE',  ( 66.89036333300305159, 144.4373801540182569, -2.303882249869787291 ) ) ;
#12168=CARTESIAN_POINT ( 'NONE',  ( 33.24893159794274311, 146.2783277815063059, 4.518043653832040540 ) ) ;
#12181=CARTESIAN_POINT ( 'NONE',  ( 43.01140435219951996, 119.9070776186055838, 50.00000000000002842 ) ) ;
#12187=CARTESIAN_POINT ( 'NONE',  ( 24.80496442426440140, 98.26638142913259344, 0.1995735771552373528 ) ) ;
#12192=CARTESIAN_POINT ( 'NONE',  ( 8.944919112598912037, 123.2842988173194385, -4.803623532975393573 ) ) ;
#12195=CARTESIAN_POINT ( 'NONE',  ( 51.29519266978688563, 92.95216133272363379, 14.08499220319455780 ) ) ;
#12196=DIRECTION ( 'NONE',  ( -0.7067093775913380060, 0.7073806645723110798, -0.01320799052465155242 ) ) ;
#12201=B_SPLINE_CURVE_WITH_KNOTS ( 'NONE', 3,
 ( #21304, #17651, #4535, #1345, #17867, #11255, #20977, #19755, #19528, #12808, #4649, #2996, #11368, #11042, #9519, #9625, #21195, #6081, #9735, #5865, #12919, #14562, #12596, #4215, #2558, #17758, #16324, #9295, #7651, #19644, #21091, #1128, #5972, #12700, #2660, #19421, #7756, #4422 ),
 .UNSPECIFIED., .F., .F.,
 ( 4, 2, 2, 2, 2, 2, 2, 2, 2, 2, 2, 2, 2, 2, 2, 2, 2, 2, 4 ),
 ( 0.01567185795944685614, 0.01665109603395603308, 0.01763033410846520654, 0.01811995314571980542, 0.01860957218297440430, 0.01958881025748360205, 0.02056804833199280327, 0.02154728640650200797, 0.02252652448101120919, 0.02350576255552041388, 0.02448500063002961857, 0.02546423870453881980, 0.02644347677904802449, 0.02693309581630264071, 0.02742271485355725694, 0.02840195292806652061, 0.02938119100257578775, 0.03036042907708504796, 0.03133966715159431510 ),
 .UNSPECIFIED. ) ;
#12206=CARTESIAN_POINT ( 'NONE',  ( 20.63953418349755253, 94.10117616956034681, -11.87063135391590052 ) ) ;
#12216=CARTESIAN_POINT ( 'NONE',  ( 70.62757080055673953, 99.67629488849819097, 13.29148015538516425 ) ) ;
#12223=CARTESIAN_POINT ( 'NONE',  ( 14.82355424275916000, 117.6079223783217458, 15.08068057431173870 ) ) ;
#12225=( LENGTH_UNIT ( ) NAMED_UNIT ( * ) SI_UNIT ( .MILLI., .METRE. ) );
#12236=CARTESIAN_POINT ( 'NONE',  ( 23.35610682547305927, 99.68565781958278649, 15.27541961222430444 ) ) ;
#12239=CARTESIAN_POINT ( 'NONE',  ( 46.06326223953917065, 144.7216122669715332, 30.23659822568390965 ) ) ;
#12249=CARTESIAN_POINT ( 'NONE',  ( 8.867590775667826719, 116.4845415224344833, 7.977433149383395872 ) ) ;
#12254=CARTESIAN_POINT ( 'NONE',  ( 67.39040179371399120, 143.9404232637865562, 4.720051584306741432 ) ) ;
#12256=CARTESIAN_POINT ( 'NONE',  ( 15.53003795322992353, 126.2325256570730687, 2.418278830334454899 ) ) ;
#12259=CARTESIAN_POINT ( 'NONE',  ( 43.01140435219952707, 144.9070776186055696, 39.21067981925356349 ) ) ;
#12263=CARTESIAN_POINT ( 'NONE',  ( 47.30009524607925897, 85.94413156685014599, 0.1962900075584997628 ) ) ;
#12274=ORIENTED_EDGE ( 'NONE', *, *, #14566, .T. ) ;
#12278=CARTESIAN_POINT ( 'NONE',  ( 65.51498131554875215, 136.7693945797108199, 5.946615082358765569 ) ) ;
#12294=CARTESIAN_POINT ( 'NONE',  ( 26.46568392313936968, 149.8720644322279725, 23.30118661649528633 ) ) ;
#12300=CARTESIAN_POINT ( 'NONE',  ( 19.03178791447554374, 95.58698510358173905, 9.200771007679692914 ) ) ;
#12301=CARTESIAN_POINT ( 'NONE',  ( 21.71662816054514167, 101.4213758857254675, 8.370706496969875232 ) ) ;
#12313=CARTESIAN_POINT ( 'NONE',  ( 11.38715737009742668, 107.0096734253407362, 2.652989958896663225 ) ) ;
#12323=CARTESIAN_POINT ( 'NONE',  ( 31.47436479266152531, 87.67613096727390598, 14.72005176623422606 ) ) ;
#12329=CARTESIAN_POINT ( 'NONE',  ( 55.65775942066846937, 145.2030105016711445, 10.43785198868815023 ) ) ;
#12341=CARTESIAN_POINT ( 'NONE',  ( 28.97945247615869846, 95.53788343559241980, -5.005900276531492388 ) ) ;
#12347=CARTESIAN_POINT ( 'NONE',  ( 46.06149648801706320, 95.09233299183981103, 38.18604851697274682 ) ) ;
#12355=CARTESIAN_POINT ( 'NONE',  ( 47.52490801233957995, 85.89149910694642642, 6.191896081848653921 ) ) ;
#12362=CARTESIAN_POINT ( 'NONE',  ( 70.85748824340309682, 124.3570181999574515, -1.510321027129504889 ) ) ;
#12368=CARTESIAN_POINT ( 'NONE',  ( 73.32203938827501588, 103.9946350594383517, -0.8753108214479579097 ) ) ;
#12383=CARTESIAN_POINT ( 'NONE',  ( 20.91437931538276374, 145.9617080342048894, -10.94665030085253044 ) ) ;
#12390=CARTESIAN_POINT ( 'NONE',  ( 19.47480796662762970, 104.5210170170265229, 9.517959287447121497 ) ) ;
#12395=EDGE_CURVE ( 'NONE', #12901, #19172, #1329, .T. ) ;
#12408=CARTESIAN_POINT ( 'NONE',  ( 34.25380259335813093, 93.01594701623474748, 13.77127495354717190 ) ) ;
#12415=CARTESIAN_POINT ( 'NONE',  ( 27.91901995959459271, 89.26896823883201648, 8.843372880480211862 ) ) ;
#12416=CARTESIAN_POINT ( 'NONE',  ( 71.07552608251525328, 117.1481954606975791, 12.77539325861266484 ) ) ;
#12427=CARTESIAN_POINT ( 'NONE',  ( 51.97100187899584967, 152.8641821122263309, -1.870631353872792335 ) ) ;
#12429=CARTESIAN_POINT ( 'NONE',  ( 62.84376099716368458, 92.00366499689042143, 13.64888190966157566 ) ) ;
#12436=CARTESIAN_POINT ( 'NONE',  ( 54.37136329154349568, 152.2862128563062072, 3.215626235130811583 ) ) ;
#12442=CARTESIAN_POINT ( 'NONE',  ( 24.99951789580824268, 141.7104366081036346, 16.15213770299339657 ) ) ;
#12453=CARTESIAN_POINT ( 'NONE',  ( 54.97053026609068382, 94.45704024927961484, -6.077358488390353308 ) ) ;
#12465=CARTESIAN_POINT ( 'NONE',  ( 67.29571637068438861, 144.1510613573267108, 10.71565575886252297 ) ) ;
#12472=CARTESIAN_POINT ( 'NONE',  ( 14.88799800344823154, 117.8296896831652560, 9.085076399755989129 ) ) ;
#12483=CARTESIAN_POINT ( 'NONE',  ( 18.20936163119166196, 143.5026679720446907, 2.934308097026923967 ) ) ;
#12493=CARTESIAN_POINT ( 'NONE',  ( 69.27296957579615366, 97.94681810169329594, -0.6368323762655749842 ) ) ;
#12500=CARTESIAN_POINT ( 'NONE',  ( 19.07518309319397432, 143.9976739860571229, -17.03742665657317801 ) ) ;
#12502=FACE_OUTER_BOUND ( 'NONE', #13290, .T. ) ;
#12520=CARTESIAN_POINT ( 'NONE',  ( 70.90273821555796019, 124.5833669296562931, 4.485287862780372947 ) ) ;
#12525=CARTESIAN_POINT ( 'NONE',  ( 69.71972837475884432, 98.49221204361529658, -7.660766391518695428 ) ) ;
#12526=CARTESIAN_POINT ( 'NONE',  ( 66.10898071834657230, 103.7292514542787245, 6.347102411281516865 ) ) ;
#12530=EDGE_LOOP ( 'NONE', ( #14715, #11407 ) ) ;
#12535=CARTESIAN_POINT ( 'NONE',  ( 21.10625685842435928, 146.1099207202125854, -2.942173209646314014 ) ) ;
#12537=CARTESIAN_POINT ( 'NONE',  ( 75.59501567365037999, 109.4093883240155378, 12.93430809701916750 ) ) ;
#12543=CARTESIAN_POINT ( 'NONE',  ( 23.80922038702690102, 91.46939207759763235, 0.001460074241615882690 ) ) ;
#12551=CARTESIAN_POINT ( 'NONE',  ( 64.86034851325717909, 101.9512479430583625, 5.437578391810254708 ) ) ;
#12562=CARTESIAN_POINT ( 'NONE',  ( 60.50179475597519740, 141.9260456451392827, -8.339099203377070779 ) ) ;
#12570=CARTESIAN_POINT ( 'NONE',  ( 61.61057083318216598, 91.16763906547615193, -7.303593892219363504 ) ) ;
#12577=CARTESIAN_POINT ( 'NONE',  ( 77.28446211531542076, 118.2294073780637262, 4.644197663618684579 ) ) ;
#12585=CARTESIAN_POINT ( 'NONE',  ( 62.59245796673033624, 99.61375035622579333, -0.4388640268946644718 ) ) ;
#12595=CARTESIAN_POINT ( 'NONE',  ( 11.39584491653312526, 106.7788786240791978, 8.648593811254444930 ) ) ;
#12596=CARTESIAN_POINT ( 'NONE',  ( 38.26722257261177873, 95.36101971774161257, 35.82300994916139558 ) ) ;
#12603=CARTESIAN_POINT ( 'NONE',  ( 32.31036143884366396, 152.4250368413922274, -10.51794503956956817 ) ) ;
#12627=CARTESIAN_POINT ( 'NONE',  ( 65.02109649036992778, 137.6666368931563227, 10.91413209638136728 ) ) ;
#12634=CARTESIAN_POINT ( 'NONE',  ( 26.90790578767411390, 150.1165885900122987, 3.291480155758420345 ) ) ;
#12635=CARTESIAN_POINT ( 'NONE',  ( 34.40470276422951912, 146.6778736915268553, -16.43444041970612446 ) ) ;
#12645=CARTESIAN_POINT ( 'NONE',  ( 14.34121205894687456, 138.4663445754194697, 3.724531598165178092 ) ) ;
#12652=CARTESIAN_POINT ( 'NONE',  ( 20.33033954036769941, 94.15838586645493535, 7.144317217164116052 ) ) ;
#12657=AXIS2_PLACEMENT_3D ( 'NONE', #2403, #7050, #17169 ) ;
#12660=CARTESIAN_POINT ( 'NONE',  ( 67.88957565821384321, 106.4565162521658976, 12.22353771717463466 ) ) ;
#12671=CARTESIAN_POINT ( 'NONE',  ( 16.34080065753823163, 110.9948608346959276, -11.19624206051981474 ) ) ;
#12673=CYLINDRICAL_SURFACE ( 'NONE', #21022, 2.999999999999997780 ) ;
#12677=CARTESIAN_POINT ( 'NONE',  ( 33.56091001181424360, 87.00402361476987778, -6.351118090676544981 ) ) ;
#12682=CARTESIAN_POINT ( 'NONE',  ( 37.02312590732701381, 153.6946607573816834, 9.644493012478044136 ) ) ;
#12690=CARTESIAN_POINT ( 'NONE',  ( 15.80414578680225723, 112.4924633436790344, 15.87081086175909306 ) ) ;
#12698=CARTESIAN_POINT ( 'NONE',  ( 63.41425016244589585, 92.41789933959738335, 6.624947895572852019 ) ) ;
#12700=CARTESIAN_POINT ( 'NONE',  ( 41.39091152515459271, 94.95783073190082746, 38.95199156105032046 ) ) ;
#12709=CARTESIAN_POINT ( 'NONE',  ( 51.60797029699607918, 86.77139250312444574, -6.946567135388369785 ) ) ;
#12715=EDGE_CURVE ( 'NONE', #17523, #3649, #13295, .T. ) ;
#12734=CARTESIAN_POINT ( 'NONE',  ( 62.80402591640378773, 99.70611228127967252, 5.556743651330835476 ) ) ;
#12740=CARTESIAN_POINT ( 'NONE',  ( 76.92284642892752800, 124.5854180935290714, 5.434424407683230207 ) ) ;
#12742=CARTESIAN_POINT ( 'NONE',  ( 31.57890723221301599, 145.5991046824261446, -16.55366158474257432 ) ) ;
#12743=CARTESIAN_POINT ( 'NONE',  ( 76.20123706073158587, 111.5182621349952257, -8.137091297256032973 ) ) ;
#12753=CARTESIAN_POINT ( 'NONE',  ( 70.84804472268019992, 100.1183116193850964, 0.2719452077637916076 ) ) ;
#12760=CARTESIAN_POINT ( 'NONE',  ( 17.52475135776945336, 142.8823211630961794, 1.906181796079885027 ) ) ;
#12766=CARTESIAN_POINT ( 'NONE',  ( 25.76509531087978289, 97.49384569152056201, 21.15186415193267067 ) ) ;
#12777=CARTESIAN_POINT ( 'NONE',  ( 22.37680805599060818, 139.0098026693046336, -10.00581381704545514 ) ) ;
#12785=CARTESIAN_POINT ( 'NONE',  ( 57.94507594753278568, 150.7106492751291569, -2.660852849641732298 ) ) ;
#12793=CARTESIAN_POINT ( 'NONE',  ( 53.94306145151312393, 87.38125778962682944, 12.97772928308168616 ) ) ;
#12807=CARTESIAN_POINT ( 'NONE',  ( 72.33162239183086228, 137.5781058455011703, 11.98183203572534872 ) ) ;
#12808=CARTESIAN_POINT ( 'NONE',  ( 39.95954646485986927, 95.09254297023964853, 30.23659822568392386 ) ) ;
#12816=CARTESIAN_POINT ( 'NONE',  ( 61.61057083318216598, 91.16763906547615193, -7.303593892219363504 ) ) ;
#12823=ORIENTED_EDGE ( 'NONE', *, *, #14589, .T. ) ;
#12841=CARTESIAN_POINT ( 'NONE',  ( 24.55476856798156859, 141.3345980244743885, 9.128255474432329208 ) ) ;
#12847=CARTESIAN_POINT ( 'NONE',  ( 69.27296957579615366, 97.94681810169329594, -0.6368323762655749842 ) ) ;
#12848=CARTESIAN_POINT ( 'NONE',  ( 60.50179475597519740, 141.9260456451392827, -8.339099203377070779 ) ) ;
#12855=AXIS2_PLACEMENT_3D ( 'NONE', #844, #15933, #12196 ) ;
#12858=CARTESIAN_POINT ( 'NONE',  ( 76.37589548207274959, 127.2077353526990748, 6.343625931721379452 ) ) ;
#12861=CARTESIAN_POINT ( 'NONE',  ( 11.08170843061617816, 132.1625483722078513, 16.49545033792581350 ) ) ;
#12869=CARTESIAN_POINT ( 'NONE',  ( 9.529548018246485341, 127.4200721877477491, 8.334841288026581196 ) ) ;
#12875=CARTESIAN_POINT ( 'NONE',  ( 69.45715107853048664, 110.1171555912624740, -7.938611875467805667 ) ) ;
#12887=CARTESIAN_POINT ( 'NONE',  ( 70.97434162403952485, 116.9407273601718202, 6.779784368693626995 ) ) ;
#12889=CARTESIAN_POINT ( 'NONE',  ( 47.07948156226018455, 144.5740439970474824, 37.12229684998504808 ) ) ;
#12896=CARTESIAN_POINT ( 'NONE',  ( 17.73005198514846725, 142.9879744078657779, -4.089424278207452801 ) ) ;
#12901=VERTEX_POINT ( 'NONE', #17777 ) ;
#12904=CARTESIAN_POINT ( 'NONE',  ( 76.78854507624612324, 113.8604396784633508, 11.78705480642107517 ) ) ;
#12908=CARTESIAN_POINT ( 'NONE',  ( 17.93535261252752022, 143.0936276526352913, -10.08503035249478685 ) ) ;
#12918=CARTESIAN_POINT ( 'NONE',  ( 67.39040179371399120, 143.9404232637865562, 4.720051584306741432 ) ) ;
#12919=CARTESIAN_POINT ( 'NONE',  ( 38.04344971605643622, 95.40557500842271565, 34.86345644064632410 ) ) ;
#12929=CARTESIAN_POINT ( 'NONE',  ( 40.02721236285810136, 85.80382532021769748, 0.4343372985580923329 ) ) ;
#12937=FILL_AREA_STYLE_COLOUR ( '', #11144 ) ;
#12954=CARTESIAN_POINT ( 'NONE',  ( 16.41399813444308364, 129.5198218381110564, 15.55674365125313763 ) ) ;
#12959=FACE_OUTER_BOUND ( 'NONE', #7525, .T. ) ;
#12960=CARTESIAN_POINT ( 'NONE',  ( 26.13368487350976110, 90.12329638092472806, 0.9106621812756837686 ) ) ;
#12962=CARTESIAN_POINT ( 'NONE',  ( 60.04598833032897431, 142.2798636455802921, -15.36278432740704147 ) ) ;
#12966=ORIENTED_EDGE ( 'NONE', *, *, #19622, .T. ) ;
#12980=CARTESIAN_POINT ( 'NONE',  ( 9.691656460246418803, 128.1079710775123601, 15.35877872671195910 ) ) ;
#12988=CARTESIAN_POINT ( 'NONE',  ( 14.76087776054169787, 121.2312262212812755, 22.22355758277721804 ) ) ;
#12999=CARTESIAN_POINT ( 'NONE',  ( 51.06471579629997137, 92.96554497763615643, 8.089385107838625188 ) ) ;
#13005=VECTOR ( 'NONE', #14259, 1000.000000000000000 ) ;
#13009=CARTESIAN_POINT ( 'NONE',  ( 75.10802748102119608, 108.0013139708956800, -8.018167963582932600 ) ) ;
#13017=CARTESIAN_POINT ( 'NONE',  ( 9.157865646370469292, 114.3054763464604662, 21.90616645148510599 ) ) ;
#13020=CARTESIAN_POINT ( 'NONE',  ( 64.37283757718545019, 93.25908544850187809, -13.41832554473225692 ) ) ;
#13023=FACE_OUTER_BOUND ( 'NONE', #395, .T. ) ;
#13024=CARTESIAN_POINT ( 'NONE',  ( 15.66613903973849986, 126.7949701480144711, 9.441967288829692606 ) ) ;
#13025=ORIENTED_EDGE ( 'NONE', *, *, #7470, .T. ) ;
#13028=CARTESIAN_POINT ( 'NONE',  ( 44.86974823489592978, 148.0457227541334362, 10.98970740178311090 ) ) ;
#13040=CARTESIAN_POINT ( 'NONE',  ( 8.798315742295939046, 121.0924013121165075, 9.124689178586496752 ) ) ;
#13063=CARTESIAN_POINT ( 'NONE',  ( 27.44638778410068625, 143.5188605762539851, 16.27111261720311930 ) ) ;
#13069=CARTESIAN_POINT ( 'NONE',  ( 24.41145734808947054, 148.6458414325078081, 10.19629000755267434 ) ) ;
#13070=CARTESIAN_POINT ( 'NONE',  ( 15.04800518778627882, 122.8738276488686694, -10.72018599084894319 ) ) ;
#13087=CARTESIAN_POINT ( 'NONE',  ( 66.46241511549931147, 94.85692098654722315, 12.50163586956050210 ) ) ;
#13095=CARTESIAN_POINT ( 'NONE',  ( 61.21858502650649569, 141.5469622553929128, 17.69968404581608823 ) ) ;
#13107=CARTESIAN_POINT ( 'NONE',  ( 15.21076168709227616, 115.6846582791190201, 9.994193321846964295 ) ) ;
#13118=CARTESIAN_POINT ( 'NONE',  ( 30.24639091383375700, 151.6717570033048048, 3.410403464249057492 ) ) ;
#13125=CARTESIAN_POINT ( 'NONE',  ( 73.16288888369128074, 103.5245705370889766, 12.14422718744263285 ) ) ;
#13128=CARTESIAN_POINT ( 'NONE',  ( 21.10625685842435928, 146.1099207202125854, -2.942173209646314014 ) ) ;
#13130=CARTESIAN_POINT ( 'NONE',  ( 22.52008984372607614, 139.2495111981779985, 17.01435058386764965 ) ) ;
#13136=CARTESIAN_POINT ( 'NONE',  ( 14.88799800344823154, 117.8296896831652560, 9.085076399755989129 ) ) ;
#13147=CARTESIAN_POINT ( 'NONE',  ( 11.67247064774405452, 106.1322524520788875, 1.624861436118421043 ) ) ;
#13153=CARTESIAN_POINT ( 'NONE',  ( 57.94507594753278568, 150.7106492751291569, -2.660852849641732298 ) ) ;
#13171=CARTESIAN_POINT ( 'NONE',  ( 31.34884810169724645, 145.5825485123889109, -10.55804779818428862 ) ) ;
#13179=CARTESIAN_POINT ( 'NONE',  ( 28.97945247615869846, 95.53788343559241980, -5.005900276531492388 ) ) ;
#13195=CARTESIAN_POINT ( 'NONE',  ( 21.21153947156776809, 146.4065673692475400, 16.07276909216647454 ) ) ;
#13200=CARTESIAN_POINT ( 'NONE',  ( 65.38231449488820601, 145.7134111962467671, 5.629255361809699210 ) ) ;
#13201=CARTESIAN_POINT ( 'NONE',  ( 30.88693878601983300, 94.35661743609990992, 20.91413290821214588 ) ) ;
#13212=CARTESIAN_POINT ( 'NONE',  ( 42.05360093099289287, 148.0107091728485500, 4.874927614337289938 ) ) ;
#13224=CARTESIAN_POINT ( 'NONE',  ( 76.92284642892752800, 124.5854180935290714, 5.434424407683230207 ) ) ;
#13232=CARTESIAN_POINT ( 'NONE',  ( 38.74908582987571748, 85.85911260889788821, 20.47761041045779606 ) ) ;
#13235=CARTESIAN_POINT ( 'NONE',  ( 10.57123148683770175, 130.5870355106474108, -10.56118268746274325 ) ) ;
#13238=AXIS2_PLACEMENT_3D ( 'NONE', #19483, #15845, #11211 ) ;
#13246=CARTESIAN_POINT ( 'NONE',  ( 21.71662816054514167, 101.4213758857254675, 8.370706496969875232 ) ) ;
#13259=CARTESIAN_POINT ( 'NONE',  ( 20.22230697948889500, 94.36241449208007737, 1.148710122009321211 ) ) ;
#13268=CARTESIAN_POINT ( 'NONE',  ( 75.85495621331871519, 129.5603373922052697, -8.732165470513974626 ) ) ;
#13270=CARTESIAN_POINT ( 'NONE',  ( 35.25059181783574758, 92.79662968204097240, -6.272318425388238694 ) ) ;
#13276=VECTOR ( 'NONE', #3656, 1000.000000000000000 ) ;
#13277=CARTESIAN_POINT ( 'NONE',  ( 9.248697603757472407, 114.7582530722838356, 9.914954709382596931 ) ) ;
#13287=CARTESIAN_POINT ( 'NONE',  ( 53.47116958538193643, 146.1823035489369715, 17.34243072007611985 ) ) ;
#13290=EDGE_LOOP ( 'NONE', ( #8205, #20115, #19435, #16756 ) ) ;
#13292=CARTESIAN_POINT ( 'NONE',  ( 8.829984022807513711, 121.7968051057545580, 16.14860047415989541 ) ) ;
#13294=CARTESIAN_POINT ( 'NONE',  ( 69.89089498905519804, 111.6491328518190613, -0.005813817042542732995 ) ) ;
#13295=CIRCLE ( 'NONE', #16094, 24.99999999999999289 ) ;
#13313=CARTESIAN_POINT ( 'NONE',  ( 59.95958160670890180, 90.07020311440788873, 19.76341270931769500 ) ) ;
#13317=CARTESIAN_POINT ( 'NONE',  ( 62.47932545177000208, 147.9683691103492436, 5.510132816154444946 ) ) ;
#13318=CARTESIAN_POINT ( 'NONE',  ( 52.49585387951581339, 146.4637788833130685, -2.700609006624497876 ) ) ;
#13330=CARTESIAN_POINT ( 'NONE',  ( 67.19681472375953035, 134.2522627023263908, 6.065787011912938453 ) ) ;
#13339=CARTESIAN_POINT ( 'NONE',  ( 40.02721236285810136, 85.80382532021769748, 0.4343372985580923329 ) ) ;
#13346=CARTESIAN_POINT ( 'NONE',  ( 16.32863300717066579, 110.5331391746388761, 0.7949662885976053195 ) ) ;
#13349=CARTESIAN_POINT ( 'NONE',  ( 20.63953418349755253, 94.10117616956034681, -11.87063135391590052 ) ) ;
#13357=CARTESIAN_POINT ( 'NONE',  ( 54.67410106651116308, 94.23276814491528341, 6.942135068398441078 ) ) ;
#13366=ORIENTED_EDGE ( 'NONE', *, *, #21507, .F. ) ;
#13369=CARTESIAN_POINT ( 'NONE',  ( 8.869018199820361659, 117.4101421016551967, 9.005765870029716069 ) ) ;
#13371=EDGE_LOOP ( 'NONE', ( #982, #12966, #21570, #6517 ) ) ;
#13377=CARTESIAN_POINT ( 'NONE',  ( 31.34884810169724645, 145.5825485123889109, -10.55804779818428862 ) ) ;
#13382=CARTESIAN_POINT ( 'NONE',  ( 71.14040157825178312, 139.4183699182763974, -9.089337262093875935 ) ) ;
#13394=CARTESIAN_POINT ( 'NONE',  ( 19.58029209685692962, 104.0714924419353480, 21.50917333468608561 ) ) ;
#13400=CARTESIAN_POINT ( 'NONE',  ( 14.88286428391304561, 100.3963227437532595, 8.410691821786379307 ) ) ;
#13402=CARTESIAN_POINT ( 'NONE',  ( 14.95244176413730131, 118.0514569880088231, 3.089472225200239563 ) ) ;
#13418=CARTESIAN_POINT ( 'NONE',  ( 17.22388115030108224, 97.27017246186569821, 14.28717435998666296 ) ) ;
#13423=CARTESIAN_POINT ( 'NONE',  ( 51.97100187899584967, 152.8641821122263309, -1.870631353872792335 ) ) ;
#13424=CARTESIAN_POINT ( 'NONE',  ( 29.12819380265916180, 95.36133955912156068, 0.9897074016940036190 ) ) ;
#13435=CARTESIAN_POINT ( 'NONE',  ( 23.40005864183818218, 147.8691531402271835, -9.846981161663094895 ) ) ;
#13446=CARTESIAN_POINT ( 'NONE',  ( 17.60877916486148465, 96.95950790538488206, 1.267834678905774393 ) ) ;
#13454=CARTESIAN_POINT ( 'NONE',  ( 24.57236314005146838, 141.2733614120550385, -4.872173989822636386 ) ) ;
#13465=CARTESIAN_POINT ( 'NONE',  ( 20.99626426110969390, 137.5292218135913913, 9.918250401459649979 ) ) ;
#13472=CARTESIAN_POINT ( 'NONE',  ( 40.50423473544901753, 144.7825417035512601, 38.54896506029345460 ) ) ;
#13477=CARTESIAN_POINT ( 'NONE',  ( 77.31131846045057898, 118.9338434746808844, -2.379532457331845485 ) ) ;
#13479=ADVANCED_BREP_SHAPE_REPRESENTATION ( '', ( #14549, #353, #12657 ), #19020 ) ;
#13484=CARTESIAN_POINT ( 'NONE',  ( 23.23160898551418185, 147.7622765488190453, -10.85157364460736140 ) ) ;
#13486=CARTESIAN_POINT ( 'NONE',  ( 52.49585387951581339, 146.4637788833130685, -2.700609006624497876 ) ) ;
#13493=CARTESIAN_POINT ( 'NONE',  ( 65.38231449488820601, 145.7134111962467671, 5.629255361809699210 ) ) ;
#13502=CARTESIAN_POINT ( 'NONE',  ( 15.50679444821833819, 113.6848169819070193, -5.081469017220888063 ) ) ;
#13508=CARTESIAN_POINT ( 'NONE',  ( 22.46358530849972723, 92.52609567587644790, 8.053519324161520387 ) ) ;
#13511=CARTESIAN_POINT ( 'NONE',  ( 16.71508173162657229, 129.8698440624217483, 3.565528294796503683 ) ) ;
#13524=CARTESIAN_POINT ( 'NONE',  ( 38.74908582987571748, 85.85911260889788821, 20.47761041045779606 ) ) ;
#13528=CARTESIAN_POINT ( 'NONE',  ( 77.16427934405430733, 119.9933672671919851, 6.581674455321548933 ) ) ;
#13529=CARTESIAN_POINT ( 'NONE',  ( 16.16443657470430750, 128.5343009702184816, -4.486436360144259616 ) ) ;
#13539=CARTESIAN_POINT ( 'NONE',  ( 75.83902229129397199, 129.3300604911257778, -14.72777435697347137 ) ) ;
#13547=CARTESIAN_POINT ( 'NONE',  ( 48.17517050666977241, 153.7480039124125994, 4.005852979123367241 ) ) ;
#13555=CARTESIAN_POINT ( 'NONE',  ( 34.49559591455799534, 146.8750064778945728, 2.580435534661669195 ) ) ;
#13564=CARTESIAN_POINT ( 'NONE',  ( 52.12662541604375122, 146.5080492276505311, -15.72009227599853531 ) ) ;
#13578=CARTESIAN_POINT ( 'NONE',  ( 31.47436479266152531, 87.67613096727390598, 14.72005176623422606 ) ) ;
#13584=CARTESIAN_POINT ( 'NONE',  ( 61.76154402333882132, 148.5480768402654803, 4.482004293238171400 ) ) ;
#13586=( NAMED_UNIT ( * ) PLANE_ANGLE_UNIT ( ) SI_UNIT ( $, .RADIAN. ) );
#13593=CARTESIAN_POINT ( 'NONE',  ( 34.64294707643933435, 153.0196542278736729, 4.557659493426334585 ) ) ;
#13603=CARTESIAN_POINT ( 'NONE',  ( 18.86999673272213229, 105.3337293714367604, -5.438779171309367833 ) ) ;
#13611=CARTESIAN_POINT ( 'NONE',  ( 28.48261614285185672, 95.83124311379776827, 2.017784757223194170 ) ) ;
#13626=CARTESIAN_POINT ( 'NONE',  ( 12.26432857192422432, 135.0705202968918570, 22.59931835930844457 ) ) ;
#13627=CARTESIAN_POINT ( 'NONE',  ( 30.18028515090310293, 151.2280014487710957, 17.43780275515693390 ) ) ;
#13632=CARTESIAN_POINT ( 'NONE',  ( 66.03587854725165585, 94.68079322629401418, 0.5104136635535641009 ) ) ;
#13633=CARTESIAN_POINT ( 'NONE',  ( 66.49460585200260709, 135.5194395740885511, -1.986604139701473759 ) ) ;
#13646=CARTESIAN_POINT ( 'NONE',  ( 54.88857506304572809, 87.88569651147935247, -13.06129575545291210 ) ) ;
#13650=DIRECTION ( 'NONE',  ( -0.7067093775913396714, 0.7073806645723093034, -0.01320799052465169467 ) ) ;
#13656=CARTESIAN_POINT ( 'NONE',  ( 32.07966263401961982, 152.4337125855422528, -4.522337938825778281 ) ) ;
#13662=CARTESIAN_POINT ( 'NONE',  ( 35.43645570112151688, 92.65990651318493576, -0.2767073223962682738 ) ) ;
#13674=CARTESIAN_POINT ( 'NONE',  ( 71.10646316465144423, 118.7373161137383732, -14.29152813157908319 ) ) ;
#13679=CARTESIAN_POINT ( 'NONE',  ( 44.30846152966199725, 94.93869211110843764, 39.05053369627938054 ) ) ;
#13686=CARTESIAN_POINT ( 'NONE',  ( 11.08170843061617816, 132.1625483722078513, 16.49545033792581350 ) ) ;
#13693=CARTESIAN_POINT ( 'NONE',  ( 37.24990543953586553, 153.6521207556136517, 3.648881909465930828 ) ) ;
#13696=( NAMED_UNIT ( * ) SI_UNIT ( $, .STERADIAN. ) SOLID_ANGLE_UNIT ( ) );
#13701=CARTESIAN_POINT ( 'NONE',  ( 9.616596702810701558, 112.3753283828585694, -5.161025107254184618 ) ) ;
#13705=( BOUNDED_SURFACE ( )  B_SPLINE_SURFACE ( 3, 3, ( 
 ( #15975, #2755, #19297, #7625, #4295, #7943, #17953, #19616, #14326, #19505, #481, #6161, #14216, #6277, #4511, #5839, #9495, #11234, #13009, #21282, #2859, #21068, #12570, #16193, #4195, #2537, #2137, #12677, #15577, #1104, #10923, #10524, #11131, #17220, #8869, #7839, #11022, #16086, #17846, #9602, #12896, #996, #17630, #7734, #14435, #16302, #21169, #6059, #12785, #4398, #10146, #21614, #16633, #6739, #19962, #18065, #11451, #18409, #16517, #16848, #3085, #18296, #6624, #18179, #1544, #13339, #9710, #4732, #11674, #2132, #13446, #15209, #20076, #1763, #8055, #6391, #11786, #4846, #6504, #14975, #109, #9819, #13118, #11342, #8163, #13547, #8497, #14869, #19841, #1433, #18516, #1653, #6841, #13224, #4622, #11567, #2971, #16412, #3198, #20181, #8385, #5072, #16742, #1321, #14761, #3426, #21503, #9928, #15094, #3309, #8275, #21721, #4964, #10038, #7273, #5596, #20713, #13975, #12106, #18838, #3961, #15629, #3638, #9032, #1977, #7383, #10363, #2193, #18625, #20283, #5489, #10255, #17279, #326, #5390, #5178, #3744, #12216, #16957, #8924, #18950, #20389, #10474, #534, #17174, #12323, #19058, #10683, #17388, #2087, #8820, #2292, #15743, #17064, #648, #8711, #11896, #15430, #3530, #1869, #8599, #3851 ),
 ( #15529, #15319, #212, #6949, #13656, #5286, #12000, #18733, #7056, #13761, #20501, #434, #7165, #13868, #20606, #19481, #2407, #5812, #5711, #19271, #19162, #4372, #15843, #2834, #14409, #11209, #4481, #11103, #9251, #12543, #21145, #7811, #6030, #861, #1185, #17925, #4271, #14517, #16168, #7598, #12760, #9573, #19588, #14297, #10999, #1080, #21041, #12436, #20931, #17816, #4171, #16279, #10900, #5924, #16057, #17604, #17709, #968, #4061, #14191, #2729, #9469, #21257, #20820, #7709, #10790, #17496, #754, #6137, #12652, #19376, #2614, #9143, #2510, #7489, #9352, #12869, #16824, #20153, #11422, #9685, #1294, #15066, #4936, #5045, #9795, #11756, #6363, #18487, #3393, #21472, #3279, #11646, #10009, #20049, #10117, #11314, #16714, #7919, #13087, #1623, #18378, #8355, #21803, #14622, #18038, #6711, #21359, #19704, #13418, #6594, #8029, #21584, #6250, #6474, #12980, #4595, #2943, #16382, #13195, #19928, #14736, #19815, #4704, #18148, #3055, #16488, #1405, #8134, #14837, #4816, #14948, #11539, #18266, #3170, #9899, #16601, #1517, #21695, #8247, #13313, #5150, #13949, #17252, #13524, #409, #10551, #3930, #5465, #15604, #6922, #3505, #7139, #11869, #15292, #15179, #13626, #6818, #13843, #10228, #12294, #2064 ),
 ( #20687, #19032, #512, #7249, #5571, #5365, #10661, #5260, #3614, #20579, #20365, #15507, #16930, #11977, #17039, #1736, #8902, #2165, #18707, #10446, #8471, #12082, #301, #18812, #1846, #20258, #18601, #8681, #10336, #3825, #12187, #18922, #7030, #8576, #81, #15403, #185, #1951, #3717, #13735, #20473, #17148, #8793, #1052, #4038, #16027, #7786, #16144, #17686, #19245, #14382, #19139, #9328, #10765, #12520, #2484, #19349, #17471, #2381, #9119, #12734, #17578, #4144, #14490, #15817, #940, #21232, #6111, #2588, #10877, #21121, #731, #7685, #7459, #9226, #15924, #4247, #14168, #20901, #5788, #12841, #836, #7570, #9443, #14270, #15717, #2269, #21015, #10973, #5897, #12627, #11075, #19559, #6005, #4454, #19457, #4347, #17790, #17363, #2698, #9006, #621, #7356, #14059, #20793, #5685, #12408, #6686, #11512, #6337, #14814, #21672, #4682, #18121, #18012, #9549, #12954, #1492, #6567, #16465, #13063, #14923, #2811, #4569, #9658, #11624, #13287, #21559, #18352, #19677, #11185, #1269, #21447, #9986, #19790, #11291, #16252, #16573, #8108, #20022, #1597, #3143, #19903, #4908, #1161, #17898, #8004, #8330, #15039, #13394, #3256, #16689, #21780, #6449, #20128, #14711, #11397, #8222, #16358, #9873, #2923, #3031 ),
 ( #9768, #7894, #1379, #13171, #4791, #18241, #14596, #21336, #6223, #6795, #8657, #5338, #12055, #13816, #10312, #382, #1712, #15152, #17122, #15266, #11845, #15379, #53, #18574, #8554, #7111, #2034, #18786, #3481, #17014, #3689, #18682, #13603, #3584, #13502, #16799, #8447, #163, #10205, #10417, #20446, #13710, #20340, #10092, #20556, #6896, #272, #20234, #1921, #16908, #8766, #5235, #1820, #15481, #5127, #7006, #5439, #5022, #11731, #11952, #18464, #3367, #16652, #18085, #19863, #9838, #4867, #2991, #9732, #16429, #17, #11470, #1341, #16762, #14888, #1230, #9622, #16538, #11588, #4750, #14781, #18429, #5091, #11364, #8405, #8075, #6648, #21524, #15114, #1454, #11694, #3327, #8187, #1673, #6299, #16321, #21411, #20198, #3216, #18199, #6525, #13357, #3106, #21634, #6413, #7964, #4646, #14998, #20094, #13246, #19982, #4983, #14671, #13136, #18316, #10056, #6757, #9949, #13465, #1564, #2883, #8291, #21740, #11805, #13028, #19752, #1783, #2101, #15445, #5506, #8941, #10489, #5404, #20623, #10168, #3443, #15338, #15647, #551, #13994, #10593, #2210, #17298, #346, #5618, #230, #20407, #8839, #12236, #3870, #18967, #7295, #10382, #17082, #20730, #13884, #1885, #18536, #6968, #16869, #8619, #450 ),
 ( #5305, #3654, #8517, #1996, #17189, #15230, #128, #6857, #13564, #20300, #5198, #15545, #11915, #18645, #7180, #3547, #13674, #10272, #16975, #12017, #18751, #8727, #7075, #13778, #20517, #12121, #18854, #3762, #9486, #2747, #9371, #7508, #10810, #12671, #6051, #19391, #14208, #21274, #16185, #2530, #12777, #14427, #20947, #4288, #1097, #17837, #5829, #9266, #21162, #12562, #3977, #19181, #11015, #2422, #7831, #17513, #4188, #14317, #4080, #15966, #21060, #17406, #12453, #17726, #7725, #19498, #14533, #5941, #12341, #15759, #14102, #4390, #19289, #10916, #878, #19076, #9162, #20838, #10702, #15861, #2311, #9050, #774, #5729, #17622, #11122, #16076, #664, #7615, #7401, #2631, #987, #10026, #19720, #1532, #9915, #8264, #18285, #16731, #9593, #14964, #1641, #17943, #16622, #4834, #6266, #19830, #21711, #4720, #16294, #4611, #19608, #11332, #11224, #11557, #7935, #8374, #6492, #3298, #18398, #3187, #1311, #18053, #13212, #6614, #19949, #8046, #15084, #6152, #18165, #13330, #20066, #14751, #4953, #12887, #11661, #21492, #3073, #4501, #6378, #2849, #12999, #1200, #2961, #14639, #9700, #11440, #8152, #16400, #9811, #14857, #21380, #13107, #16506, #1423, #21603, #10568, #1967, #18941, #3414, #1754, #7155 ),
 ( #8489, #20490, #5481, #20595, #7045, #1860, #18828, #15198, #5380, #101, #16944, #6939, #8700, #6832, #13539, #20274, #3841, #8590, #5166, #13858, #11991, #20173, #6729, #13646, #15421, #15309, #11887, #15520, #2180, #18615, #12206, #3520, #3733, #10246, #17269, #20380, #8809, #423, #18721, #15495, #10137, #13435, #18505, #5063, #12095, #201, #3628, #10463, #10352, #17055, #17164, #11776, #2078, #16841, #4264, #20921, #17488, #19366, #7264, #9023, #14075, #16048, #10992, #19262, #959, #17378, #15619, #5703, #4054, #14400, #2718, #19473, #5804, #9345, #17702, #2398, #853, #4365, #21138, #10782, #12535, #2607, #9135, #13965, #639, #7589, #12427, #6022, #20813, #7481, #17596, #7374, #4164, #2502, #20705, #15734, #14289, #7702, #12753, #11095, #9244, #17807, #19049, #2283, #527, #15835, #746, #10893, #5588, #19153, #14183, #12313, #15943, #3949, #10675, #21033, #5916, #12645, #16897, #6784, #6886, #11615, #13593, #8213, #20331, #5228, #1176, #5117, #13493, #11835, #44, #11943, #12858, #18565, #18673, #21250, #20225, #8433, #9565, #1589, #3471, #8320, #10195, #1811, #8543, #15255, #15030, #21770, #154, #9459, #14912, #16160, #13277, #1072, #21662, #7802, #14508, #6128, #16791, #19579, #4472, #18343 ),
 ( #11202, #17915, #2825, #16270, #6552, #15141, #20012, #4896, #3244, #9975, #16679, #6675, #13382, #20120, #5011, #11720, #18455, #3356, #10081, #1704, #14127, #3898, #691, #15785, #580, #20547, #2027, #10622, #19107, #17330, #5430, #20652, #12048, #262, #13701, #10520, #15474, #5648, #14023, #7323, #2130, #15369, #20866, #17215, #8971, #6997, #5535, #8757, #20757, #3791, #12150, #9078, #18778, #2237, #7428, #2341, #15676, #18882, #12368, #5330, #4003, #3681, #8865, #15573, #12263, #10409, #17111, #374, #5753, #477, #7104, #17433, #7213, #1911, #10301, #13913, #18998, #10732, #13809, #12483, #3575, #17004, #8647, #20436, #1127, #4214, #2886, #4317, #6187, #12918, #2659, #17975, #800, #4107, #15887, #14673, #4421, #14349, #1019, #7861, #12698, #11041, #10943, #17539, #20976, #9518, #14561, #9403, #21090, #21303, #10843, #12595, #17650, #19643, #4534, #14454, #11254, #5864, #19210, #9294, #7650, #9624, #5971, #19316, #2449, #2778, #16113, #16323, #1232, #11151, #12807, #7966, #9189, #7534, #15995, #21414, #6302, #14236, #2557, #904, #19420, #21193, #17757, #17866, #16217, #18431, #18201, #4986, #21526, #3108, #6528, #10171, #20200, #19, #9840, #21743, #6759, #1567, #11590, #19867, #11696, #16540 ) ),
 .UNSPECIFIED., .T., .F., .F. ) 
 B_SPLINE_SURFACE_WITH_KNOTS ( ( 4, 3, 4 ),
 ( 4, 2, 2, 2, 2, 2, 2, 2, 2, 2, 2, 2, 2, 2, 2, 2, 2, 2, 2, 2, 2, 2, 2, 2, 2, 2, 2, 2, 2, 2, 2, 2, 2, 2, 2, 2, 2, 2, 2, 2, 2, 2, 2, 2, 2, 2, 2, 2, 2, 2, 2, 2, 2, 2, 2, 2, 2, 2, 2, 2, 2, 2, 2, 2, 2, 2, 2, 2, 2, 2, 2, 2, 2, 2, 2, 2, 2, 2, 2, 2, 4 ),
 ( 0.000000000000000000, 0.5000000000000000000, 1.000000000000000000 ),
 ( 0.000000000000000000, 0.008318061648474830982, 0.01871563870907547167, 0.02911321576967611582, 0.03951079283027675998, 0.04990836989087740067, 0.06030594695147804829, 0.07070352401207868898, 0.08110110107267932966, 0.09149867813327997035, 0.1018962551938805972, 0.1122938322544812378, 0.1226914093150818785, 0.1330889863756825053, 0.1434865634362831321, 0.1538841404968837590, 0.1642817175574843858, 0.1746792946180850126, 0.1850768716786856394, 0.1954744487392862939, 0.2058720257998869485, 0.2162696028604875753, 0.2266671799210882021, 0.2370647569816888289, 0.2474623340422894557, 0.2578599111028900825, 0.2682574881634907094, 0.2786550652240913362, 0.2890526422846919630, 0.2994502193452925343, 0.3098477964058931611, 0.3202453734664937879, 0.3306429505270944147, 0.3410405275876950415, 0.3514381046482956683, 0.3618356817088962951, 0.3722332587694969219, 0.3826308358300975487, 0.3930284128906983421, 0.4034259899512990799, 0.4138235670118998732, 0.4242211440725006666, 0.4346187211331002942, 0.4450162981936999218, 0.4554138752542995494, 0.4658114523148991770, 0.4762090293755006920, 0.4866066064361021515, 0.4970041834967036110, 0.5074017605573051259, 0.5177993376179057528, 0.5281969146785063796, 0.5385944917391070064, 0.5489920687997077442, 0.5593896458603083710, 0.5697872229209089978, 0.5801847999815096246, 0.5905823770421102514, 0.6009799541027108782, 0.6113775311633115050, 0.6217751082239121319, 0.6321726852845127587, 0.6425702623451133855, 0.6529678394057140123, 0.6633654164663146391, 0.6737629935269152659, 0.6841605705875142274, 0.6945581476481130778, 0.7049557247087120393, 0.7153533017693110008, 0.7257508788299132929, 0.7361484558905155851, 0.7465460329511179882, 0.7569436100117202804, 0.7673411870723210182, 0.7777387641329216450, 0.7881363411935222718, 0.7985339182541228986, 0.8080132075800156022, 0.8174924969059083057, 0.8280181261579530050 ),
 .UNSPECIFIED. ) 
 GEOMETRIC_REPRESENTATION_ITEM ( )  RATIONAL_B_SPLINE_SURFACE ( (
 ( 1.000000000000000000, 1.000000000000000000, 1.000000000000000000, 1.000000000000000000, 1.000000000000000000, 1.000000000000000000, 1.000000000000000000, 1.000000000000000000, 1.000000000000000000, 1.000000000000000000, 1.000000000000000000, 1.000000000000000000, 1.000000000000000000, 1.000000000000000000, 1.000000000000000000, 1.000000000000000000, 1.000000000000000000, 1.000000000000000000, 1.000000000000000000, 1.000000000000000000, 1.000000000000000000, 1.000000000000000000, 1.000000000000000000, 1.000000000000000000, 1.000000000000000000, 1.000000000000000000, 1.000000000000000000, 1.000000000000000000, 1.000000000000000000, 1.000000000000000000, 1.000000000000000000, 1.000000000000000000, 1.000000000000000000, 1.000000000000000000, 1.000000000000000000, 1.000000000000000000, 1.000000000000000000, 1.000000000000000000, 1.000000000000000000, 1.000000000000000000, 1.000000000000000000, 1.000000000000000000, 1.000000000000000000, 1.000000000000000000, 1.000000000000000000, 1.000000000000000000, 1.000000000000000000, 1.000000000000000000, 1.000000000000000000, 1.000000000000000000, 1.000000000000000000, 1.000000000000000000, 1.000000000000000000, 1.000000000000000000, 1.000000000000000000, 1.000000000000000000, 1.000000000000000000, 1.000000000000000000, 1.000000000000000000, 1.000000000000000000, 1.000000000000000000, 1.000000000000000000, 1.000000000000000000, 1.000000000000000000, 1.000000000000000000, 1.000000000000000000, 1.000000000000000000, 1.000000000000000000, 1.000000000000000000, 1.000000000000000000, 1.000000000000000000, 1.000000000000000000, 1.000000000000000000, 1.000000000000000000, 1.000000000000000000, 1.000000000000000000, 1.000000000000000000, 1.000000000000000000, 1.000000000000000000, 1.000000000000000000, 1.000000000000000000, 1.000000000000000000, 1.000000000000000000, 1.000000000000000000, 1.000000000000000000, 1.000000000000000000, 1.000000000000000000, 1.000000000000000000, 1.000000000000000000, 1.000000000000000000, 1.000000000000000000, 1.000000000000000000, 1.000000000000000000, 1.000000000000000000, 1.000000000000000000, 1.000000000000000000, 1.000000000000000000, 1.000000000000000000, 1.000000000000000000, 1.000000000000000000, 1.000000000000000000, 1.000000000000000000, 1.000000000000000000, 1.000000000000000000, 1.000000000000000000, 1.000000000000000000, 1.000000000000000000, 1.000000000000000000, 1.000000000000000000, 1.000000000000000000, 1.000000000000000000, 1.000000000000000000, 1.000000000000000000, 1.000000000000000000, 1.000000000000000000, 1.000000000000000000, 1.000000000000000000, 1.000000000000000000, 1.000000000000000000, 1.000000000000000000, 1.000000000000000000, 1.000000000000000000, 1.000000000000000000, 1.000000000000000000, 1.000000000000000000, 1.000000000000000000, 1.000000000000000000, 1.000000000000000000, 1.000000000000000000, 1.000000000000000000, 1.000000000000000000, 1.000000000000000000, 1.000000000000000000, 1.000000000000000000, 1.000000000000000000, 1.000000000000000000, 1.000000000000000000, 1.000000000000000000, 1.000000000000000000, 1.000000000000000000, 1.000000000000000000, 1.000000000000000000, 1.000000000000000000, 1.000000000000000000, 1.000000000000000000, 1.000000000000000000, 1.000000000000000000, 1.000000000000000000, 1.000000000000000000, 1.000000000000000000, 1.000000000000000000, 1.000000000000000000, 1.000000000000000000, 1.000000000000000000, 1.000000000000000000, 1.000000000000000000, 1.000000000000000000, 1.000000000000000000, 1.000000000000000000, 1.000000000000000000, 1.000000000000000000, 1.000000000000000000),
 ( 0.3333333333333333703, 0.3333333333333333703, 0.3333333333333333703, 0.3333333333333333703, 0.3333333333333333703, 0.3333333333333333703, 0.3333333333333333703, 0.3333333333333333703, 0.3333333333333333703, 0.3333333333333333703, 0.3333333333333333703, 0.3333333333333333703, 0.3333333333333333703, 0.3333333333333333703, 0.3333333333333333703, 0.3333333333333333703, 0.3333333333333333703, 0.3333333333333333703, 0.3333333333333333703, 0.3333333333333333703, 0.3333333333333333703, 0.3333333333333333703, 0.3333333333333333703, 0.3333333333333333703, 0.3333333333333333703, 0.3333333333333333703, 0.3333333333333333703, 0.3333333333333333703, 0.3333333333333333703, 0.3333333333333333703, 0.3333333333333333703, 0.3333333333333333703, 0.3333333333333333703, 0.3333333333333333703, 0.3333333333333333703, 0.3333333333333333703, 0.3333333333333333703, 0.3333333333333333703, 0.3333333333333333703, 0.3333333333333333703, 0.3333333333333333703, 0.3333333333333333703, 0.3333333333333333703, 0.3333333333333333703, 0.3333333333333333703, 0.3333333333333333703, 0.3333333333333333703, 0.3333333333333333703, 0.3333333333333333703, 0.3333333333333333703, 0.3333333333333333703, 0.3333333333333333703, 0.3333333333333333703, 0.3333333333333333703, 0.3333333333333333703, 0.3333333333333333703, 0.3333333333333333703, 0.3333333333333333703, 0.3333333333333333703, 0.3333333333333333703, 0.3333333333333333703, 0.3333333333333333703, 0.3333333333333333703, 0.3333333333333333703, 0.3333333333333333703, 0.3333333333333333703, 0.3333333333333333703, 0.3333333333333333703, 0.3333333333333333703, 0.3333333333333333703, 0.3333333333333333703, 0.3333333333333333703, 0.3333333333333333703, 0.3333333333333333703, 0.3333333333333333703, 0.3333333333333333703, 0.3333333333333333703, 0.3333333333333333703, 0.3333333333333333703, 0.3333333333333333703, 0.3333333333333333703, 0.3333333333333333703, 0.3333333333333333703, 0.3333333333333333703, 0.3333333333333333703, 0.3333333333333333703, 0.3333333333333333703, 0.3333333333333333703, 0.3333333333333333703, 0.3333333333333333703, 0.3333333333333333703, 0.3333333333333333703, 0.3333333333333333703, 0.3333333333333333703, 0.3333333333333333703, 0.3333333333333333703, 0.3333333333333333703, 0.3333333333333333703, 0.3333333333333333703, 0.3333333333333333703, 0.3333333333333333703, 0.3333333333333333703, 0.3333333333333333703, 0.3333333333333333703, 0.3333333333333333703, 0.3333333333333333703, 0.3333333333333333703, 0.3333333333333333703, 0.3333333333333333703, 0.3333333333333333703, 0.3333333333333333703, 0.3333333333333333703, 0.3333333333333333703, 0.3333333333333333703, 0.3333333333333333703, 0.3333333333333333703, 0.3333333333333333703, 0.3333333333333333703, 0.3333333333333333703, 0.3333333333333333703, 0.3333333333333333703, 0.3333333333333333703, 0.3333333333333333703, 0.3333333333333333703, 0.3333333333333333703, 0.3333333333333333703, 0.3333333333333333703, 0.3333333333333333703, 0.3333333333333333703, 0.3333333333333333703, 0.3333333333333333703, 0.3333333333333333703, 0.3333333333333333703, 0.3333333333333333703, 0.3333333333333333703, 0.3333333333333333703, 0.3333333333333333703, 0.3333333333333333703, 0.3333333333333333703, 0.3333333333333333703, 0.3333333333333333703, 0.3333333333333333703, 0.3333333333333333703, 0.3333333333333333703, 0.3333333333333333703, 0.3333333333333333703, 0.3333333333333333703, 0.3333333333333333703, 0.3333333333333333703, 0.3333333333333333703, 0.3333333333333333703, 0.3333333333333333703, 0.3333333333333333703, 0.3333333333333333703, 0.3333333333333333703, 0.3333333333333333703, 0.3333333333333333703, 0.3333333333333333703, 0.3333333333333333703, 0.3333333333333333703, 0.3333333333333333703, 0.3333333333333333703),
 ( 0.3333333333333333703, 0.3333333333333333703, 0.3333333333333333703, 0.3333333333333333703, 0.3333333333333333703, 0.3333333333333333703, 0.3333333333333333703, 0.3333333333333333703, 0.3333333333333333703, 0.3333333333333333703, 0.3333333333333333703, 0.3333333333333333703, 0.3333333333333333703, 0.3333333333333333703, 0.3333333333333333703, 0.3333333333333333703, 0.3333333333333333703, 0.3333333333333333703, 0.3333333333333333703, 0.3333333333333333703, 0.3333333333333333703, 0.3333333333333333703, 0.3333333333333333703, 0.3333333333333333703, 0.3333333333333333703, 0.3333333333333333703, 0.3333333333333333703, 0.3333333333333333703, 0.3333333333333333703, 0.3333333333333333703, 0.3333333333333333703, 0.3333333333333333703, 0.3333333333333333703, 0.3333333333333333703, 0.3333333333333333703, 0.3333333333333333703, 0.3333333333333333703, 0.3333333333333333703, 0.3333333333333333703, 0.3333333333333333703, 0.3333333333333333703, 0.3333333333333333703, 0.3333333333333333703, 0.3333333333333333703, 0.3333333333333333703, 0.3333333333333333703, 0.3333333333333333703, 0.3333333333333333703, 0.3333333333333333703, 0.3333333333333333703, 0.3333333333333333703, 0.3333333333333333703, 0.3333333333333333703, 0.3333333333333333703, 0.3333333333333333703, 0.3333333333333333703, 0.3333333333333333703, 0.3333333333333333703, 0.3333333333333333703, 0.3333333333333333703, 0.3333333333333333703, 0.3333333333333333703, 0.3333333333333333703, 0.3333333333333333703, 0.3333333333333333703, 0.3333333333333333703, 0.3333333333333333703, 0.3333333333333333703, 0.3333333333333333703, 0.3333333333333333703, 0.3333333333333333703, 0.3333333333333333703, 0.3333333333333333703, 0.3333333333333333703, 0.3333333333333333703, 0.3333333333333333703, 0.3333333333333333703, 0.3333333333333333703, 0.3333333333333333703, 0.3333333333333333703, 0.3333333333333333703, 0.3333333333333333703, 0.3333333333333333703, 0.3333333333333333703, 0.3333333333333333703, 0.3333333333333333703, 0.3333333333333333703, 0.3333333333333333703, 0.3333333333333333703, 0.3333333333333333703, 0.3333333333333333703, 0.3333333333333333703, 0.3333333333333333703, 0.3333333333333333703, 0.3333333333333333703, 0.3333333333333333703, 0.3333333333333333703, 0.3333333333333333703, 0.3333333333333333703, 0.3333333333333333703, 0.3333333333333333703, 0.3333333333333333703, 0.3333333333333333703, 0.3333333333333333703, 0.3333333333333333703, 0.3333333333333333703, 0.3333333333333333703, 0.3333333333333333703, 0.3333333333333333703, 0.3333333333333333703, 0.3333333333333333703, 0.3333333333333333703, 0.3333333333333333703, 0.3333333333333333703, 0.3333333333333333703, 0.3333333333333333703, 0.3333333333333333703, 0.3333333333333333703, 0.3333333333333333703, 0.3333333333333333703, 0.3333333333333333703, 0.3333333333333333703, 0.3333333333333333703, 0.3333333333333333703, 0.3333333333333333703, 0.3333333333333333703, 0.3333333333333333703, 0.3333333333333333703, 0.3333333333333333703, 0.3333333333333333703, 0.3333333333333333703, 0.3333333333333333703, 0.3333333333333333703, 0.3333333333333333703, 0.3333333333333333703, 0.3333333333333333703, 0.3333333333333333703, 0.3333333333333333703, 0.3333333333333333703, 0.3333333333333333703, 0.3333333333333333703, 0.3333333333333333703, 0.3333333333333333703, 0.3333333333333333703, 0.3333333333333333703, 0.3333333333333333703, 0.3333333333333333703, 0.3333333333333333703, 0.3333333333333333703, 0.3333333333333333703, 0.3333333333333333703, 0.3333333333333333703, 0.3333333333333333703, 0.3333333333333333703, 0.3333333333333333703, 0.3333333333333333703, 0.3333333333333333703, 0.3333333333333333703, 0.3333333333333333703, 0.3333333333333333703, 0.3333333333333333703, 0.3333333333333333703),
 ( 1.000000000000000000, 1.000000000000000000, 1.000000000000000000, 1.000000000000000000, 1.000000000000000000, 1.000000000000000000, 1.000000000000000000, 1.000000000000000000, 1.000000000000000000, 1.000000000000000000, 1.000000000000000000, 1.000000000000000000, 1.000000000000000000, 1.000000000000000000, 1.000000000000000000, 1.000000000000000000, 1.000000000000000000, 1.000000000000000000, 1.000000000000000000, 1.000000000000000000, 1.000000000000000000, 1.000000000000000000, 1.000000000000000000, 1.000000000000000000, 1.000000000000000000, 1.000000000000000000, 1.000000000000000000, 1.000000000000000000, 1.000000000000000000, 1.000000000000000000, 1.000000000000000000, 1.000000000000000000, 1.000000000000000000, 1.000000000000000000, 1.000000000000000000, 1.000000000000000000, 1.000000000000000000, 1.000000000000000000, 1.000000000000000000, 1.000000000000000000, 1.000000000000000000, 1.000000000000000000, 1.000000000000000000, 1.000000000000000000, 1.000000000000000000, 1.000000000000000000, 1.000000000000000000, 1.000000000000000000, 1.000000000000000000, 1.000000000000000000, 1.000000000000000000, 1.000000000000000000, 1.000000000000000000, 1.000000000000000000, 1.000000000000000000, 1.000000000000000000, 1.000000000000000000, 1.000000000000000000, 1.000000000000000000, 1.000000000000000000, 1.000000000000000000, 1.000000000000000000, 1.000000000000000000, 1.000000000000000000, 1.000000000000000000, 1.000000000000000000, 1.000000000000000000, 1.000000000000000000, 1.000000000000000000, 1.000000000000000000, 1.000000000000000000, 1.000000000000000000, 1.000000000000000000, 1.000000000000000000, 1.000000000000000000, 1.000000000000000000, 1.000000000000000000, 1.000000000000000000, 1.000000000000000000, 1.000000000000000000, 1.000000000000000000, 1.000000000000000000, 1.000000000000000000, 1.000000000000000000, 1.000000000000000000, 1.000000000000000000, 1.000000000000000000, 1.000000000000000000, 1.000000000000000000, 1.000000000000000000, 1.000000000000000000, 1.000000000000000000, 1.000000000000000000, 1.000000000000000000, 1.000000000000000000, 1.000000000000000000, 1.000000000000000000, 1.000000000000000000, 1.000000000000000000, 1.000000000000000000, 1.000000000000000000, 1.000000000000000000, 1.000000000000000000, 1.000000000000000000, 1.000000000000000000, 1.000000000000000000, 1.000000000000000000, 1.000000000000000000, 1.000000000000000000, 1.000000000000000000, 1.000000000000000000, 1.000000000000000000, 1.000000000000000000, 1.000000000000000000, 1.000000000000000000, 1.000000000000000000, 1.000000000000000000, 1.000000000000000000, 1.000000000000000000, 1.000000000000000000, 1.000000000000000000, 1.000000000000000000, 1.000000000000000000, 1.000000000000000000, 1.000000000000000000, 1.000000000000000000, 1.000000000000000000, 1.000000000000000000, 1.000000000000000000, 1.000000000000000000, 1.000000000000000000, 1.000000000000000000, 1.000000000000000000, 1.000000000000000000, 1.000000000000000000, 1.000000000000000000, 1.000000000000000000, 1.000000000000000000, 1.000000000000000000, 1.000000000000000000, 1.000000000000000000, 1.000000000000000000, 1.000000000000000000, 1.000000000000000000, 1.000000000000000000, 1.000000000000000000, 1.000000000000000000, 1.000000000000000000, 1.000000000000000000, 1.000000000000000000, 1.000000000000000000, 1.000000000000000000, 1.000000000000000000, 1.000000000000000000, 1.000000000000000000, 1.000000000000000000, 1.000000000000000000, 1.000000000000000000, 1.000000000000000000, 1.000000000000000000, 1.000000000000000000, 1.000000000000000000),
 ( 0.3333333333333333703, 0.3333333333333333703, 0.3333333333333333703, 0.3333333333333333703, 0.3333333333333333703, 0.3333333333333333703, 0.3333333333333333703, 0.3333333333333333703, 0.3333333333333333703, 0.3333333333333333703, 0.3333333333333333703, 0.3333333333333333703, 0.3333333333333333703, 0.3333333333333333703, 0.3333333333333333703, 0.3333333333333333703, 0.3333333333333333703, 0.3333333333333333703, 0.3333333333333333703, 0.3333333333333333703, 0.3333333333333333703, 0.3333333333333333703, 0.3333333333333333703, 0.3333333333333333703, 0.3333333333333333703, 0.3333333333333333703, 0.3333333333333333703, 0.3333333333333333703, 0.3333333333333333703, 0.3333333333333333703, 0.3333333333333333703, 0.3333333333333333703, 0.3333333333333333703, 0.3333333333333333703, 0.3333333333333333703, 0.3333333333333333703, 0.3333333333333333703, 0.3333333333333333703, 0.3333333333333333703, 0.3333333333333333703, 0.3333333333333333703, 0.3333333333333333703, 0.3333333333333333703, 0.3333333333333333703, 0.3333333333333333703, 0.3333333333333333703, 0.3333333333333333703, 0.3333333333333333703, 0.3333333333333333703, 0.3333333333333333703, 0.3333333333333333703, 0.3333333333333333703, 0.3333333333333333703, 0.3333333333333333703, 0.3333333333333333703, 0.3333333333333333703, 0.3333333333333333703, 0.3333333333333333703, 0.3333333333333333703, 0.3333333333333333703, 0.3333333333333333703, 0.3333333333333333703, 0.3333333333333333703, 0.3333333333333333703, 0.3333333333333333703, 0.3333333333333333703, 0.3333333333333333703, 0.3333333333333333703, 0.3333333333333333703, 0.3333333333333333703, 0.3333333333333333703, 0.3333333333333333703, 0.3333333333333333703, 0.3333333333333333703, 0.3333333333333333703, 0.3333333333333333703, 0.3333333333333333703, 0.3333333333333333703, 0.3333333333333333703, 0.3333333333333333703, 0.3333333333333333703, 0.3333333333333333703, 0.3333333333333333703, 0.3333333333333333703, 0.3333333333333333703, 0.3333333333333333703, 0.3333333333333333703, 0.3333333333333333703, 0.3333333333333333703, 0.3333333333333333703, 0.3333333333333333703, 0.3333333333333333703, 0.3333333333333333703, 0.3333333333333333703, 0.3333333333333333703, 0.3333333333333333703, 0.3333333333333333703, 0.3333333333333333703, 0.3333333333333333703, 0.3333333333333333703, 0.3333333333333333703, 0.3333333333333333703, 0.3333333333333333703, 0.3333333333333333703, 0.3333333333333333703, 0.3333333333333333703, 0.3333333333333333703, 0.3333333333333333703, 0.3333333333333333703, 0.3333333333333333703, 0.3333333333333333703, 0.3333333333333333703, 0.3333333333333333703, 0.3333333333333333703, 0.3333333333333333703, 0.3333333333333333703, 0.3333333333333333703, 0.3333333333333333703, 0.3333333333333333703, 0.3333333333333333703, 0.3333333333333333703, 0.3333333333333333703, 0.3333333333333333703, 0.3333333333333333703, 0.3333333333333333703, 0.3333333333333333703, 0.3333333333333333703, 0.3333333333333333703, 0.3333333333333333703, 0.3333333333333333703, 0.3333333333333333703, 0.3333333333333333703, 0.3333333333333333703, 0.3333333333333333703, 0.3333333333333333703, 0.3333333333333333703, 0.3333333333333333703, 0.3333333333333333703, 0.3333333333333333703, 0.3333333333333333703, 0.3333333333333333703, 0.3333333333333333703, 0.3333333333333333703, 0.3333333333333333703, 0.3333333333333333703, 0.3333333333333333703, 0.3333333333333333703, 0.3333333333333333703, 0.3333333333333333703, 0.3333333333333333703, 0.3333333333333333703, 0.3333333333333333703, 0.3333333333333333703, 0.3333333333333333703, 0.3333333333333333703, 0.3333333333333333703, 0.3333333333333333703, 0.3333333333333333703, 0.3333333333333333703, 0.3333333333333333703, 0.3333333333333333703, 0.3333333333333333703),
 ( 0.3333333333333333703, 0.3333333333333333703, 0.3333333333333333703, 0.3333333333333333703, 0.3333333333333333703, 0.3333333333333333703, 0.3333333333333333703, 0.3333333333333333703, 0.3333333333333333703, 0.3333333333333333703, 0.3333333333333333703, 0.3333333333333333703, 0.3333333333333333703, 0.3333333333333333703, 0.3333333333333333703, 0.3333333333333333703, 0.3333333333333333703, 0.3333333333333333703, 0.3333333333333333703, 0.3333333333333333703, 0.3333333333333333703, 0.3333333333333333703, 0.3333333333333333703, 0.3333333333333333703, 0.3333333333333333703, 0.3333333333333333703, 0.3333333333333333703, 0.3333333333333333703, 0.3333333333333333703, 0.3333333333333333703, 0.3333333333333333703, 0.3333333333333333703, 0.3333333333333333703, 0.3333333333333333703, 0.3333333333333333703, 0.3333333333333333703, 0.3333333333333333703, 0.3333333333333333703, 0.3333333333333333703, 0.3333333333333333703, 0.3333333333333333703, 0.3333333333333333703, 0.3333333333333333703, 0.3333333333333333703, 0.3333333333333333703, 0.3333333333333333703, 0.3333333333333333703, 0.3333333333333333703, 0.3333333333333333703, 0.3333333333333333703, 0.3333333333333333703, 0.3333333333333333703, 0.3333333333333333703, 0.3333333333333333703, 0.3333333333333333703, 0.3333333333333333703, 0.3333333333333333703, 0.3333333333333333703, 0.3333333333333333703, 0.3333333333333333703, 0.3333333333333333703, 0.3333333333333333703, 0.3333333333333333703, 0.3333333333333333703, 0.3333333333333333703, 0.3333333333333333703, 0.3333333333333333703, 0.3333333333333333703, 0.3333333333333333703, 0.3333333333333333703, 0.3333333333333333703, 0.3333333333333333703, 0.3333333333333333703, 0.3333333333333333703, 0.3333333333333333703, 0.3333333333333333703, 0.3333333333333333703, 0.3333333333333333703, 0.3333333333333333703, 0.3333333333333333703, 0.3333333333333333703, 0.3333333333333333703, 0.3333333333333333703, 0.3333333333333333703, 0.3333333333333333703, 0.3333333333333333703, 0.3333333333333333703, 0.3333333333333333703, 0.3333333333333333703, 0.3333333333333333703, 0.3333333333333333703, 0.3333333333333333703, 0.3333333333333333703, 0.3333333333333333703, 0.3333333333333333703, 0.3333333333333333703, 0.3333333333333333703, 0.3333333333333333703, 0.3333333333333333703, 0.3333333333333333703, 0.3333333333333333703, 0.3333333333333333703, 0.3333333333333333703, 0.3333333333333333703, 0.3333333333333333703, 0.3333333333333333703, 0.3333333333333333703, 0.3333333333333333703, 0.3333333333333333703, 0.3333333333333333703, 0.3333333333333333703, 0.3333333333333333703, 0.3333333333333333703, 0.3333333333333333703, 0.3333333333333333703, 0.3333333333333333703, 0.3333333333333333703, 0.3333333333333333703, 0.3333333333333333703, 0.3333333333333333703, 0.3333333333333333703, 0.3333333333333333703, 0.3333333333333333703, 0.3333333333333333703, 0.3333333333333333703, 0.3333333333333333703, 0.3333333333333333703, 0.3333333333333333703, 0.3333333333333333703, 0.3333333333333333703, 0.3333333333333333703, 0.3333333333333333703, 0.3333333333333333703, 0.3333333333333333703, 0.3333333333333333703, 0.3333333333333333703, 0.3333333333333333703, 0.3333333333333333703, 0.3333333333333333703, 0.3333333333333333703, 0.3333333333333333703, 0.3333333333333333703, 0.3333333333333333703, 0.3333333333333333703, 0.3333333333333333703, 0.3333333333333333703, 0.3333333333333333703, 0.3333333333333333703, 0.3333333333333333703, 0.3333333333333333703, 0.3333333333333333703, 0.3333333333333333703, 0.3333333333333333703, 0.3333333333333333703, 0.3333333333333333703, 0.3333333333333333703, 0.3333333333333333703, 0.3333333333333333703, 0.3333333333333333703, 0.3333333333333333703, 0.3333333333333333703, 0.3333333333333333703),
 ( 1.000000000000000000, 1.000000000000000000, 1.000000000000000000, 1.000000000000000000, 1.000000000000000000, 1.000000000000000000, 1.000000000000000000, 1.000000000000000000, 1.000000000000000000, 1.000000000000000000, 1.000000000000000000, 1.000000000000000000, 1.000000000000000000, 1.000000000000000000, 1.000000000000000000, 1.000000000000000000, 1.000000000000000000, 1.000000000000000000, 1.000000000000000000, 1.000000000000000000, 1.000000000000000000, 1.000000000000000000, 1.000000000000000000, 1.000000000000000000, 1.000000000000000000, 1.000000000000000000, 1.000000000000000000, 1.000000000000000000, 1.000000000000000000, 1.000000000000000000, 1.000000000000000000, 1.000000000000000000, 1.000000000000000000, 1.000000000000000000, 1.000000000000000000, 1.000000000000000000, 1.000000000000000000, 1.000000000000000000, 1.000000000000000000, 1.000000000000000000, 1.000000000000000000, 1.000000000000000000, 1.000000000000000000, 1.000000000000000000, 1.000000000000000000, 1.000000000000000000, 1.000000000000000000, 1.000000000000000000, 1.000000000000000000, 1.000000000000000000, 1.000000000000000000, 1.000000000000000000, 1.000000000000000000, 1.000000000000000000, 1.000000000000000000, 1.000000000000000000, 1.000000000000000000, 1.000000000000000000, 1.000000000000000000, 1.000000000000000000, 1.000000000000000000, 1.000000000000000000, 1.000000000000000000, 1.000000000000000000, 1.000000000000000000, 1.000000000000000000, 1.000000000000000000, 1.000000000000000000, 1.000000000000000000, 1.000000000000000000, 1.000000000000000000, 1.000000000000000000, 1.000000000000000000, 1.000000000000000000, 1.000000000000000000, 1.000000000000000000, 1.000000000000000000, 1.000000000000000000, 1.000000000000000000, 1.000000000000000000, 1.000000000000000000, 1.000000000000000000, 1.000000000000000000, 1.000000000000000000, 1.000000000000000000, 1.000000000000000000, 1.000000000000000000, 1.000000000000000000, 1.000000000000000000, 1.000000000000000000, 1.000000000000000000, 1.000000000000000000, 1.000000000000000000, 1.000000000000000000, 1.000000000000000000, 1.000000000000000000, 1.000000000000000000, 1.000000000000000000, 1.000000000000000000, 1.000000000000000000, 1.000000000000000000, 1.000000000000000000, 1.000000000000000000, 1.000000000000000000, 1.000000000000000000, 1.000000000000000000, 1.000000000000000000, 1.000000000000000000, 1.000000000000000000, 1.000000000000000000, 1.000000000000000000, 1.000000000000000000, 1.000000000000000000, 1.000000000000000000, 1.000000000000000000, 1.000000000000000000, 1.000000000000000000, 1.000000000000000000, 1.000000000000000000, 1.000000000000000000, 1.000000000000000000, 1.000000000000000000, 1.000000000000000000, 1.000000000000000000, 1.000000000000000000, 1.000000000000000000, 1.000000000000000000, 1.000000000000000000, 1.000000000000000000, 1.000000000000000000, 1.000000000000000000, 1.000000000000000000, 1.000000000000000000, 1.000000000000000000, 1.000000000000000000, 1.000000000000000000, 1.000000000000000000, 1.000000000000000000, 1.000000000000000000, 1.000000000000000000, 1.000000000000000000, 1.000000000000000000, 1.000000000000000000, 1.000000000000000000, 1.000000000000000000, 1.000000000000000000, 1.000000000000000000, 1.000000000000000000, 1.000000000000000000, 1.000000000000000000, 1.000000000000000000, 1.000000000000000000, 1.000000000000000000, 1.000000000000000000, 1.000000000000000000, 1.000000000000000000, 1.000000000000000000, 1.000000000000000000, 1.000000000000000000, 1.000000000000000000, 1.000000000000000000, 1.000000000000000000) ) ) 
 REPRESENTATION_ITEM ( '' )  SURFACE ( )  );
#13710=CARTESIAN_POINT ( 'NONE',  ( 26.65597624659334031, 142.8797025615743337, -3.772066457372480475 ) ) ;
#13715=VERTEX_POINT ( 'NONE', #21188 ) ;
#13719=CARTESIAN_POINT ( 'NONE',  ( 59.14563986918259531, 96.87627350248034475, 7.732070471200789719 ) ) ;
#13724=B_SPLINE_CURVE_WITH_KNOTS ( 'NONE', 3,
 ( #11713, #15020, #13484, #6013, #18448, #11492, #15134, #3346, #10074, #14498, #4886, #16783, #6543, #16557, #13268, #4355, #14391, #12743, #3125, #7794, #1694, #6668, #1472, #19465, #20216, #9855, #1583, #11084, #20002, #1062, #8425, #18219, #19883, #5109, #17798, #16671, #17694, #2596, #18335, #4771, #9335, #16035, #949, #2709, #8204, #16152, #21241, #6119, #13153, #14905, #21654, #11607, #3236, #9968, #15666, #15248, #7200, #569, #1803, #15564, #10509, #14014, #20321, #17318, #11933, #467, #18664, #2228, #18770, #20642, #5525, #17101, #10612, #146, #18558, #8536, #7313, #12139, #6989, #15465, #13903, #6877, #2121, #13693, #3671, #20747, #10401, #3780, #13584, #12254, #3463, #11825, #10187, #5220, #17205, #18985, #16889, #3889, #8959, #16994, #3568, #10292, #20427, #1903, #8638, #8857, #15360, #12039, #251, #2017, #20536, #5323, #8748, #366, #7093, #13798, #5422, #18873, #17811, #9463, #2722, #15945, #19475, #6024, #5806, #10994, #14511, #16163, #20924, #855, #1075, #7376, #5705, #11098, #19266, #12537, #14291, #21252, #9137, #12429, #10677, #7805, #6132, #4266, #4166, #961, #19155, #17704, #4056, #10895, #17598, #5919, #10784, #17491, #2401, #12861, #2504, #15837, #3951, #7592, #2286, #21140 ),
 .UNSPECIFIED., .F., .F.,
 ( 4, 2, 2, 2, 2, 2, 2, 2, 2, 2, 2, 2, 2, 2, 2, 2, 2, 2, 2, 2, 2, 2, 2, 2, 2, 2, 2, 2, 2, 2, 2, 2, 2, 2, 2, 2, 2, 2, 2, 2, 2, 2, 2, 2, 2, 2, 2, 2, 2, 2, 2, 2, 2, 2, 2, 2, 2, 2, 2, 2, 2, 2, 2, 2, 2, 2, 2, 2, 2, 2, 2, 2, 2, 2, 2, 2, 2, 2, 2, 2, 4 ),
 ( 0.000000000000000000, 0.008318061648474830982, 0.01871563870907547167, 0.02911321576967611582, 0.03951079283027675998, 0.04990836989087740067, 0.06030594695147804829, 0.07070352401207868898, 0.08110110107267932966, 0.09149867813327997035, 0.1018962551938806110, 0.1122938322544812378, 0.1226914093150818785, 0.1330889863756825053, 0.1434865634362831321, 0.1538841404968837590, 0.1642817175574844135, 0.1746792946180850126, 0.1850768716786856394, 0.1954744487392862939, 0.2058720257998869485, 0.2162696028604875753, 0.2266671799210882021, 0.2370647569816888289, 0.2474623340422894557, 0.2578599111028900825, 0.2682574881634907094, 0.2786550652240913362, 0.2890526422846919630, 0.2994502193452925343, 0.3098477964058931611, 0.3202453734664938434, 0.3306429505270944147, 0.3410405275876950415, 0.3514381046482956683, 0.3618356817088962951, 0.3722332587694969219, 0.3826308358300975487, 0.3930284128906983421, 0.4034259899512990799, 0.4138235670118998732, 0.4242211440725006666, 0.4346187211331003497, 0.4450162981936999218, 0.4554138752542995494, 0.4658114523148991770, 0.4762090293755007475, 0.4866066064361022070, 0.4970041834967036110, 0.5074017605573051259, 0.5177993376179057528, 0.5281969146785063796, 0.5385944917391070064, 0.5489920687997077442, 0.5593896458603083710, 0.5697872229209089978, 0.5801847999815096246, 0.5905823770421102514, 0.6009799541027108782, 0.6113775311633115050, 0.6217751082239121319, 0.6321726852845127587, 0.6425702623451133855, 0.6529678394057140123, 0.6633654164663146391, 0.6737629935269153769, 0.6841605705875142274, 0.6945581476481129668, 0.7049557247087120393, 0.7153533017693110008, 0.7257508788299132929, 0.7361484558905155851, 0.7465460329511179882, 0.7569436100117202804, 0.7673411870723210182, 0.7777387641329215340, 0.7881363411935222718, 0.7985339182541228986, 0.8080132075800156022, 0.8174924969059083057, 0.8280181261579530050 ),
 .UNSPECIFIED. ) ;
#13735=CARTESIAN_POINT ( 'NONE',  ( 20.05807715703862470, 136.4285572017038248, 1.866423417236719118 ) ) ;
#13740=CARTESIAN_POINT ( 'NONE',  ( 11.23391594879739941, 132.3357020601377769, 10.49983985543964415 ) ) ;
#13741=CARTESIAN_POINT ( 'NONE',  ( 37.56771007382699423, 92.23784766911828115, 0.6328166970475824771 ) ) ;
#13761=CARTESIAN_POINT ( 'NONE',  ( 60.35187701982888342, 149.5179833730722407, -3.570052342179399485 ) ) ;
#13766=CARTESIAN_POINT ( 'NONE',  ( 59.79647059797250819, 142.6686746773435459, -3.371582063846674693 ) ) ;
#13768=EDGE_CURVE ( 'NONE', #18531, #8368, #6408, .T. ) ;
#13770=EDGE_LOOP ( 'NONE', ( #9386, #5499, #6373, #287 ) ) ;
#13778=CARTESIAN_POINT ( 'NONE',  ( 52.77336176550079472, 93.53620953014643646, -12.98192714454240182 ) ) ;
#13783=CARTESIAN_POINT ( 'NONE',  ( 45.52178281274064631, 95.03194855707397437, 29.87433574750618703 ) ) ;
#13790=CARTESIAN_POINT ( 'NONE',  ( 8.829984022807513711, 121.7968051057545580, 16.14860047415989541 ) ) ;
#13795=AXIS2_PLACEMENT_3D ( 'NONE', #7280, #7496, #14197 ) ;
#13798=CARTESIAN_POINT ( 'NONE',  ( 9.822352152143091431, 128.2981216602131553, 9.363167623699879982 ) ) ;
#13801=CARTESIAN_POINT ( 'NONE',  ( 65.09246388851926213, 137.4469437283422906, 4.918530982704383270 ) ) ;
#13809=CARTESIAN_POINT ( 'NONE',  ( 13.78455932396994577, 137.7305411390292420, 2.696406107442721467 ) ) ;
#13816=CARTESIAN_POINT ( 'NONE',  ( 69.04633063039527485, 130.7408809369782716, -8.772150750671475095 ) ) ;
#13827=CARTESIAN_POINT ( 'NONE',  ( 23.25700774553339301, 99.89415360575743819, 9.279811863844059872 ) ) ;
#13843=CARTESIAN_POINT ( 'NONE',  ( 17.92634965299622252, 143.2997274935095788, 22.91961472066619265 ) ) ;
#13849=CARTESIAN_POINT ( 'NONE',  ( 10.61900875472251649, 108.8314319666055212, -5.279948415675857376 ) ) ;
#13850=CARTESIAN_POINT ( 'NONE',  ( 71.20918238807936973, 120.1790618917378879, 12.65642078274776416 ) ) ;
#13858=CARTESIAN_POINT ( 'NONE',  ( 71.68162264554656815, 101.3460857334412708, -13.77530061520655025 ) ) ;
#13868=CARTESIAN_POINT ( 'NONE',  ( 74.61827669547474784, 133.2649018527303895, -2.855682626312802785 ) ) ;
#13874=CARTESIAN_POINT ( 'NONE',  ( 70.86003890729777766, 114.9808142912368254, 11.86642341732858874 ) ) ;
#13884=CARTESIAN_POINT ( 'NONE',  ( 16.70103016558074316, 129.9804388327498827, 16.57432765154378629 ) ) ;
#13891=CARTESIAN_POINT ( 'NONE',  ( 46.98443111744539635, 95.22409955470565990, 37.26405200954400954 ) ) ;
#13898=CARTESIAN_POINT ( 'NONE',  ( 8.916504151126011024, 123.7798070670463773, 8.215921583872152212 ) ) ;
#13903=CARTESIAN_POINT ( 'NONE',  ( 20.88913110926514705, 146.0313881486468119, 3.053432864643822686 ) ) ;
#13905=CARTESIAN_POINT ( 'NONE',  ( 68.29827362630597065, 132.3882971431532383, 5.156253003121209488 ) ) ;
#13913=CARTESIAN_POINT ( 'NONE',  ( 9.021810916323596885, 123.9851095102452945, 2.220310480865780534 ) ) ;
#13931=CARTESIAN_POINT ( 'NONE',  ( 74.95715479139145998, 107.8263973513541742, -14.01376907723217613 ) ) ;
#13949=CARTESIAN_POINT ( 'NONE',  ( 49.69400319086401652, 86.25038505451357196, 20.12058643263999969 ) ) ;
#13954=CARTESIAN_POINT ( 'NONE',  ( 12.59043673732666946, 104.3826120832696773, 9.557940159192295226 ) ) ;
#13956=CARTESIAN_POINT ( 'NONE',  ( 70.94289844336020678, 123.7826807253454575, 5.513563639855703080 ) ) ;
#13965=CARTESIAN_POINT ( 'NONE',  ( 37.47668497174467461, 153.6095807538456199, -2.346729193546184700 ) ) ;
#13975=CARTESIAN_POINT ( 'NONE',  ( 14.15704070161504369, 138.3271338521546454, 9.720138693322796897 ) ) ;
#13981=CARTESIAN_POINT ( 'NONE',  ( 58.30185729850432352, 143.6975816885063750, 10.55682690296339032 ) ) ;
#13988=EDGE_LOOP ( 'NONE', ( #2653, #1927, #5990, #18579 ) ) ;
#13994=CARTESIAN_POINT ( 'NONE',  ( 59.36841858216658352, 96.93634223693318575, 13.72768157422830981 ) ) ;
#14001=CARTESIAN_POINT ( 'NONE',  ( 46.31788101060713814, 95.12560940527907860, 37.97538637126936578 ) ) ;
#14008=CARTESIAN_POINT ( 'NONE',  ( 76.90526227772885193, 114.5556580205831096, 4.763324653225488703 ) ) ;
#14010=ORIENTED_EDGE ( 'NONE', *, *, #13768, .F. ) ;
#14012=DIRECTION ( 'NONE',  ( -0.7067093775913396714, 0.7073806645723093034, -0.01320799052465169467 ) ) ;
#14014=CARTESIAN_POINT ( 'NONE',  ( 61.01612483116806374, 90.79174121657607088, -0.2798613066081144796 ) ) ;
#14016=CARTESIAN_POINT ( 'NONE',  ( 15.00983914341701997, 123.2415857317943448, 2.299110145932334426 ) ) ;
#14023=CARTESIAN_POINT ( 'NONE',  ( 11.74529739132928619, 133.8467647624810581, -4.446451035385589279 ) ) ;
#14034=CARTESIAN_POINT ( 'NONE',  ( 77.19215121279506775, 118.0176990621192203, -1.351406188750652992 ) ) ;
#14036=ORIENTED_EDGE ( 'NONE', *, *, #3491, .F. ) ;
#14040=CARTESIAN_POINT ( 'NONE',  ( 27.04509496028088478, 143.0549882411833380, 11.23409068567602098 ) ) ;
#14059=CARTESIAN_POINT ( 'NONE',  ( 46.21245884545565019, 91.80782910428004584, 13.29499484581607582 ) ) ;
#14065=CARTESIAN_POINT ( 'NONE',  ( 23.63511980923729183, 148.0372221624750466, 11.16864677238829984 ) ) ;
#14066=CARTESIAN_POINT ( 'NONE',  ( 65.77248029998415291, 103.2585056976580091, 13.37079068582577435 ) ) ;
#14075=CARTESIAN_POINT ( 'NONE',  ( 66.55041322599720388, 95.16028120083096553, -6.513516925475251185 ) ) ;
#14090=CARTESIAN_POINT ( 'NONE',  ( 66.29928749942908439, 103.8601778506706239, 12.34270352495849110 ) ) ;
#14095=( GEOMETRIC_REPRESENTATION_CONTEXT ( 3 ) GLOBAL_UNCERTAINTY_ASSIGNED_CONTEXT ( ( #10628 ) ) GLOBAL_UNIT_ASSIGNED_CONTEXT ( ( #12225, #2621, #7716 ) ) REPRESENTATION_CONTEXT ( 'NONE', 'WORKASPACE' ) );
#14102=CARTESIAN_POINT ( 'NONE',  ( 22.01597290215339697, 101.2010103422484519, -4.648787059867797389 ) ) ;
#14113=CARTESIAN_POINT ( 'NONE',  ( 51.59368247783319816, 153.1301807948854616, 10.12058642595840929 ) ) ;
#14120=CARTESIAN_POINT ( 'NONE',  ( 69.49396330798431620, 129.5978393632817927, 5.275421687385184910 ) ) ;
#14127=CARTESIAN_POINT ( 'NONE',  ( 69.71972837475884432, 98.49221204361529658, -7.660766391518695428 ) ) ;
#14140=CARTESIAN_POINT ( 'NONE',  ( 74.85601106972485752, 107.3429126181175661, -0.9942341299615756745 ) ) ;
#14147=CARTESIAN_POINT ( 'NONE',  ( 27.89715912807487186, 143.6191053679247602, 4.279900468622926724 ) ) ;
#14158=LINE ( 'NONE', #19339, #13005 ) ;
#14168=CARTESIAN_POINT ( 'NONE',  ( 17.32321720400341292, 131.7349665092470730, 8.652027877775747555 ) ) ;
#14174=CARTESIAN_POINT ( 'NONE',  ( 50.33192209904863290, 153.3481575868430014, -9.922832680162505525 ) ) ;
#14175=CARTESIAN_POINT ( 'NONE',  ( 51.84853669763433004, 93.12814091139611605, 7.061107544354192633 ) ) ;
#14183=CARTESIAN_POINT ( 'NONE',  ( 14.82542406694137860, 100.6198891296320994, 2.415082931867933880 ) ) ;
#14191=CARTESIAN_POINT ( 'NONE',  ( 69.47322557110069852, 98.06143112153284846, 5.358778726746561638 ) ) ;
#14195=ADVANCED_FACE ( 'NONE', ( #12502 ), #603, .T. ) ;
#14197=DIRECTION ( 'NONE',  ( -0.3428981916074304581, 0.9393725726208712601, 0.000000000000000000 ) ) ;
#14199=CARTESIAN_POINT ( 'NONE',  ( 62.80402591640378773, 99.70611228127967252, 5.556743651330835476 ) ) ;
#14208=CARTESIAN_POINT ( 'NONE',  ( 15.04800518778627882, 122.8738276488686694, -10.72018599084894319 ) ) ;
#14216=CARTESIAN_POINT ( 'NONE',  ( 71.14040157825178312, 139.4183699182763974, -9.089337262093875935 ) ) ;
#14222=CARTESIAN_POINT ( 'NONE',  ( 8.843693174888816344, 123.0768258502195067, 1.191984145255910787 ) ) ;
#14228=CARTESIAN_POINT ( 'NONE',  ( 46.56541826512206228, 91.93282113015048651, 0.2755065429245392439 ) ) ;
#14236=CARTESIAN_POINT ( 'NONE',  ( 70.62757080055673953, 99.67629488849819097, 13.29148015538516425 ) ) ;
#14244=CARTESIAN_POINT ( 'NONE',  ( 17.73005198514846725, 142.9879744078657779, -4.089424278207452801 ) ) ;
#14245=DIRECTION ( 'NONE',  ( -1.000000000000000000, 0.000000000000000000, 0.000000000000000000 ) ) ;
#14249=CARTESIAN_POINT ( 'NONE',  ( 10.62509257988331335, 109.0622927966340967, -11.27555259023744405 ) ) ;
#14259=DIRECTION ( 'NONE',  ( 0.000000000000000000, 0.000000000000000000, -1.000000000000000000 ) ) ;
#14270=CARTESIAN_POINT ( 'NONE',  ( 41.03523200113699687, 148.1191603456353789, 9.842457937073838536 ) ) ;
#14276=CARTESIAN_POINT ( 'NONE',  ( 69.83118287335672392, 141.1824132108841638, 4.838974892866481525 ) ) ;
#14278=CARTESIAN_POINT ( 'NONE',  ( 70.04389262751028866, 127.6510855156269599, -14.64878692017946626 ) ) ;
#14289=CARTESIAN_POINT ( 'NONE',  ( 75.66441332552922461, 109.8968089748874064, -0.08503035249486777525 ) ) ;
#14291=CARTESIAN_POINT ( 'NONE',  ( 74.27779736592162863, 105.9683817680885056, 13.05343286460986363 ) ) ;
#14293=DIRECTION ( 'NONE',  ( -0.000000000000000000, -0.000000000000000000, -1.000000000000000000 ) ) ;
#14297=CARTESIAN_POINT ( 'NONE',  ( 32.75162935850930523, 152.6515011162663313, 2.501635869428501469 ) ) ;
#14306=CARTESIAN_POINT ( 'NONE',  ( 32.01435502045076475, 93.85226834503447435, 6.866149820358673495 ) ) ;
#14317=CARTESIAN_POINT ( 'NONE',  ( 69.09677972725788209, 109.4046064338026127, -6.910527774811301427 ) ) ;
#14320=CARTESIAN_POINT ( 'NONE',  ( 47.50216252638477954, 144.5007669503875150, 31.98784611697848135 ) ) ;
#14326=CARTESIAN_POINT ( 'NONE',  ( 53.88337135589062399, 152.3674195137575964, -9.803719146365084569 ) ) ;
#14334=CARTESIAN_POINT ( 'NONE',  ( 76.86499250339331013, 125.5074929390188316, 4.406300711698651895 ) ) ;
#14341=CARTESIAN_POINT ( 'NONE',  ( 26.83015598135647295, 142.9878415585355071, 17.22988066553158149 ) ) ;
#14349=CARTESIAN_POINT ( 'NONE',  ( 72.98789752971651978, 103.3738663174133023, 6.148623012889737005 ) ) ;
#14358=CARTESIAN_POINT ( 'NONE',  ( 50.33192209904863290, 153.3481575868430014, -9.922832680162505525 ) ) ;
#14379=SHAPE_DEFINITION_REPRESENTATION ( #16436, #14632 ) ;
#14382=CARTESIAN_POINT ( 'NONE',  ( 62.56935518920172967, 140.3353681171158200, 3.771274953561639887 ) ) ;
#14388=CARTESIAN_POINT ( 'NONE',  ( 53.71239221804358976, 87.38980250447106357, 6.982120393166105998 ) ) ;
#14389=CARTESIAN_POINT ( 'NONE',  ( 22.37680805599060818, 139.0098026693046336, -10.00581381704545514 ) ) ;
#14391=CARTESIAN_POINT ( 'NONE',  ( 77.22348061889915982, 118.7203125366680752, -8.375138532479306619 ) ) ;
#14400=CARTESIAN_POINT ( 'NONE',  ( 20.11427441861009058, 94.56644311770523359, -4.846896973145477183 ) ) ;
#14409=CARTESIAN_POINT ( 'NONE',  ( 51.83766784316492249, 86.74794057323931895, -0.9509610611041249273 ) ) ;
#14416=CARTESIAN_POINT ( 'NONE',  ( 33.70380864093198170, 93.20109254516876263, 20.79496611990781929 ) ) ;
#14427=CARTESIAN_POINT ( 'NONE',  ( 26.87902611899987448, 142.9395564687116007, -9.767670631928341507 ) ) ;
#14429=CARTESIAN_POINT ( 'NONE',  ( 31.20897972572456069, 148.4098837309091721, 17.43780275515692679 ) ) ;
#14435=CARTESIAN_POINT ( 'NONE',  ( 36.55618291757107841, 153.5264344809625641, -3.375052104409746789 ) ) ;
#14441=CARTESIAN_POINT ( 'NONE',  ( 77.32109437525961937, 120.4276527761501399, 18.57288864564252506 ) ) ;
#14448=CARTESIAN_POINT ( 'NONE',  ( 29.48178659935447854, 144.5857871963822845, 17.33364154221121467 ) ) ;
#14454=CARTESIAN_POINT ( 'NONE',  ( 9.822352152143091431, 128.2981216602131553, 9.363167623699879982 ) ) ;
#14462=CARTESIAN_POINT ( 'NONE',  ( 10.42839491720816625, 130.4056617841633283, -4.565575592310756825 ) ) ;
#14463=FACE_OUTER_BOUND ( 'NONE', #11516, .T. ) ;
#14490=CARTESIAN_POINT ( 'NONE',  ( 49.77943037783704483, 92.44786530929899016, 6.152137702922222395 ) ) ;
#14496=CARTESIAN_POINT ( 'NONE',  ( 64.11693453485118255, 146.8606268255622638, -2.422805558527139080 ) ) ;
#14497=CARTESIAN_POINT ( 'NONE',  ( 52.67254683800726411, 146.3150465326280028, -8.696212858991016148 ) ) ;
#14498=CARTESIAN_POINT ( 'NONE',  ( 60.49690154327523572, 149.3382625450468311, -9.565656633516235630 ) ) ;
#14508=CARTESIAN_POINT ( 'NONE',  ( 12.60192345832597027, 135.3850619972812979, 10.60811072801600119 ) ) ;
#14511=CARTESIAN_POINT ( 'NONE',  ( 55.94180145820917716, 151.6039095241057453, 11.26783467880839140 ) ) ;
#14517=CARTESIAN_POINT ( 'NONE',  ( 10.28555834757860055, 130.2242880576791890, 1.430031502841225821 ) ) ;
#14523=CARTESIAN_POINT ( 'NONE',  ( 26.70363248220801466, 142.8423586596025245, -10.77201286955609127 ) ) ;
#14533=CARTESIAN_POINT ( 'NONE',  ( 37.37095630934955892, 92.35886976769425871, -5.362784416626555029 ) ) ;
#14535=CARTESIAN_POINT ( 'NONE',  ( 47.34826785674352578, 144.5287207813994996, 31.70117790783977796 ) ) ;
#14541=FACE_OUTER_BOUND ( 'NONE', #13988, .T. ) ;
#14549=MANIFOLD_SOLID_BREP ( 'Sweep1', #17939 ) ;
#14550=CARTESIAN_POINT ( 'NONE',  ( 72.28893465744093305, 137.8051215927966382, 17.97743314940082371 ) ) ;
#14555=CARTESIAN_POINT ( 'NONE',  ( 17.81206540393426252, 132.5069038242342003, 16.68302557436956945 ) ) ;
#14561=CARTESIAN_POINT ( 'NONE',  ( 32.14050509837299785, 87.44534670509604268, 7.696117750009315195 ) ) ;
#14562=CARTESIAN_POINT ( 'NONE',  ( 38.17059775574655589, 95.38013743195961069, 35.50423386912937218 ) ) ;
#14566=EDGE_CURVE ( 'NONE', #10804, #18715, #7260, .T. ) ;
#14570=CARTESIAN_POINT ( 'NONE',  ( 18.20936163119166196, 143.5026679720446907, 2.934308097026923967 ) ) ;
#14589=EDGE_CURVE ( 'NONE', #2680, #21236, #17313, .T. ) ;
#14595=( BOUNDED_SURFACE ( )  B_SPLINE_SURFACE ( 3, 3, ( 
 ( #7661, #12383, #2567, #4013, #12603, #4225, #10636, #14358, #17443, #2354, #7765, #19220, #9092, #2670, #809, #8981, #17340, #17550, #19325, #5765, #703, #4326, #12816, #19118, #12709, #2459, #10953, #7334, #16004, #6088, #7546, #915, #19535, #9414, #9199, #15897, #16122, #14462, #19432, #7437, #14244, #21099, #4118, #20988, #11051, #17766, #17661, #15794, #1028, #9304, #21205, #5873, #5982, #2247, #20769, #14034, #5660, #14140, #20877, #12493, #10854, #16334, #14684, #3228, #21424, #12929, #9528, #9849, #1355, #13259, #16665, #18213, #13147, #6538, #17874, #11161, #19996, #11376, #6313, #14570, #18097, #1243, #4880, #14899, #1466, #3007, #16225, #21752, #9744, #16550, #1136, #9962, #8198, #7977, #21647, #11599, #7871, #21312, #3118, #6197, #6662, #19653, #1576, #18329, #4544, #8304, #11266, #6425, #19876, #4429, #15012, #17985, #2899, #13369, #13040, #9634, #2785, #16441, #19764, #4661, #8086, #4763, #14793, #21535, #11484, #462, #6768, #359, #5213, #20420, #10068, #3665, #15558, #10284, #10395, #7194, #12134, #18656, #11927, #18867, #17200, #7087, #10180, #1896, #8742, #13578, #3560, #20530, #5416, #5317, #3457, #3775, #12030, #13790, #8632, #13686, #2115, #8417, #6983, #20106, #17095, #18764 ),
 ( #11819, #11705, #16881, #3340, #2010, #30, #8852, #15459, #4995, #10503, #18441, #20209, #16989, #16777, #1687, #15127, #13477, #20315, #5103, #15350, #18551, #1798, #140, #8529, #15242, #6870, #245, #4093, #15981, #7414, #5519, #20742, #5847, #3991, #4302, #18979, #14222, #9064, #17635, #8954, #10826, #9388, #17741, #2646, #5630, #9280, #2543, #891, #4200, #16093, #17311, #7630, #1003, #3882, #14334, #12577, #14008, #5741, #11028, #2325, #21074, #2223, #15660, #785, #12355, #15772, #19091, #2435, #563, #5956, #17525, #9174, #15873, #10716, #12249, #13898, #20962, #10607, #676, #10928, #19302, #7308, #7521, #12682, #20637, #17419, #14113, #19405, #20851, #12465, #19196, #16524, #9717, #9936, #21621, #12904, #9503, #13125, #17852, #21292, #21175, #19626, #12793, #19847, #16200, #18303, #8061, #4854, #19970, #4738, #7847, #4630, #3205, #6066, #6512, #16641, #1220, #4405, #19737, #1442, #9826, #9611, #8171, #1112, #11574, #7740, #11349, #14876, #7953, #19513, #14550, #21512, #4520, #14441, #11137, #14769, #2867, #16418, #18072, #1328, #2763, #6170, #6397, #3093, #13232, #11242, #11457, #17962, #16309, #14658, #21398, #6286, #13017, #2979, #18186, #18739, #5395, #8282, #20507, #15217, #4970, #18419 ),
 ( #1551, #13454, #11794, #332, #18524, #10046, #6633, #6955, #20290, #10369, #13766, #15326, #10261, #3642, #14983, #21728, #17069, #3433, #8504, #12112, #20083, #6746, #18843, #3750, #10479, #5080, #10155, #13662, #20188, #16856, #20396, #8716, #1770, #13346, #15434, #1983, #116, #16963, #7061, #11903, #16750, #219, #6847, #13555, #11682, #5184, #18632, #3317, #12005, #5291, #3536, #1659, #8392, #1875, #15101, #5, #8606, #20938, #7282, #12551, #14199, #440, #5495, #15849, #20612, #19381, #7170, #14306, #5818, #18956, #9151, #10583, #19169, #10798, #17179, #19277, #17285, #2200, #21048, #3967, #8930, #9256, #7391, #15534, #2093, #2298, #4069, #12329, #13981, #10907, #4276, #3858, #4178, #9040, #17501, #13874, #760, #12660, #14090, #7497, #8825, #15956, #15750, #654, #869, #5930, #17610, #20719, #20826, #2516, #10690, #5718, #7603, #12223, #2412, #540, #15636, #5604, #19065, #12442, #17396, #8141, #21152, #19710, #11005, #8035, #17930, #1086, #13095, #21481, #14743, #9581, #974, #6481, #2840, #16388, #7715, #9802, #6369, #7818, #19821, #4711, #16064, #6037, #9691, #14416, #13201, #12766, #14845, #11429, #19487, #2950, #4379, #12988, #4601, #17715, #18155, #11110, #17826, #21590, #19596, #2735 ),
 ( #11320, #6142, #14523, #3062, #19937, #9475, #16494, #16285, #18044, #16175, #1301, #2620, #1191, #1413, #9360, #21263, #7924, #14628, #12875, #4489, #11214, #21367, #6256, #15297, #20161, #11763, #5266, #11982, #5156, #10015, #18712, #11875, #6928, #8479, #20264, #1956, #14954, #13529, #4823, #1850, #18606, #16831, #11546, #16719, #15073, #3619, #21809, #13318, #9905, #10234, #1743, #13633, #17044, #3510, #16935, #20370, #18273, #3176, #10341, #6718, #18494, #8686, #1523, #1629, #15410, #307, #13741, #8362, #13424, #8581, #5051, #3399, #190, #7035, #10125, #16610, #8252, #21700, #15186, #6600, #20054, #89, #4941, #11651, #6821, #18386, #3286, #9233, #7578, #2170, #519, #4045, #17259, #13956, #10772, #5795, #20694, #17585, #12526, #7467, #8908, #7364, #14175, #9013, #7146, #19145, #5577, #15610, #8799, #12301, #10558, #739, #9125, #17480, #19041, #10452, #15932, #3937, #2389, #17153, #19252, #15824, #7255, #20909, #4154, #3723, #15512, #10884, #2070, #843, #414, #2492, #20479, #13850, #12416, #20585, #628, #14066, #5371, #12087, #5471, #12195, #18817, #10667, #18931, #3831, #17370, #2274, #15725, #20801, #5692, #9451, #4354, #8012, #16472, #948, #16366, #21240, #14604, #4254, #19685, #9777 ),
 ( #17906, #11194, #2818, #12742, #12635, #1388, #21343, #10980, #2707, #11297, #12962, #19356, #7901, #1277, #14278, #17693, #11083, #18020, #2930, #9666, #6231, #14719, #16259, #21023, #6344, #19464, #16034, #4576, #2595, #6012, #5905, #17797, #9334, #21454, #7693, #3038, #13070, #11405, #4688, #19798, #14389, #9556, #21129, #16151, #18129, #1060, #7793, #14497, #6118, #12848, #19568, #4462, #1168, #1829, #10214, #9994, #8561, #16580, #20349, #8117, #20135, #16916, #1605, #21566, #14932, #61, #20032, #5244, #13179, #8456, #3262, #10100, #5030, #16808, #19912, #8230, #15161, #3490, #15273, #18692, #1723, #11960, #11520, #9882, #21680, #1499, #4917, #6576, #6802, #173, #3593, #14821, #10320, #21788, #18250, #3150, #13294, #11630, #6905, #5136, #11853, #18359, #11739, #17022, #6457, #4798, #16698, #13611, #18583, #8337, #20244, #15049, #6695, #13402, #18472, #3375, #13511, #600, #2044, #15589, #14147, #12168, #9099, #5348, #18795, #10642, #392, #18901, #8775, #12278, #10426, #5666, #5551, #20670, #19014, #7120, #282, #10860, #8988, #13719, #3808, #20775, #7341, #7015, #17345, #10747, #19227, #20455, #13827, #12390, #19125, #4019, #2253, #17451, #3915, #4125, #15800, #20566, #3698, #14040, #12065, #15490 ),
 ( #12500, #15695, #20883, #5771, #2360, #5449, #710, #1932, #17130, #7443, #17233, #8665, #15387, #10535, #2149, #8882, #494, #7231, #13931, #16527, #2983, #13020, #6174, #9720, #7956, #19973, #6515, #14879, #16421, #7552, #13349, #1332, #1446, #14249, #16644, #21624, #14660, #13235, #4858, #815, #12908, #8174, #20994, #20086, #19630, #14986, #11577, #4523, #9828, #11245, #19851, #11461, #17558, #18305, #17966, #2871, #21731, #4633, #9614, #9938, #8066, #15904, #2465, #14772, #4741, #19741, #21403, #3208, #4973, #16313, #1554, #21515, #18189, #1223, #8285, #9205, #6400, #6639, #6289, #11353, #13128, #3097, #18075, #6926, #3509, #21699, #13423, #20262, #3284, #1628, #10233, #16934, #10124, #14953, #8579, #16829, #11874, #20160, #3398, #13632, #19936, #18493, #9800, #6820, #1742, #21808, #16493, #6599, #20053, #15296, #11650, #18271, #14844, #15185, #6717, #189, #20369, #8478, #87, #5265, #1412, #8139, #18711, #18385, #8361, #21589, #6480, #13317, #13200, #4821, #11545, #10014, #15072, #13528, #5050, #11761, #5155, #3175, #9904, #16608, #1522, #8251, #10771, #18929, #738, #17478, #12415, #413, #12300, #19144, #13954, #12086, #2273, #10556, #20584, #13740, #17258, #15511, #5691, #14065, #627, #2169 ),
 ( #18816, #7145, #3721, #3936, #20800, #7466, #10340, #14174, #8907, #7034, #20477, #5370, #10450, #2388, #7362, #4044, #17152, #15609, #20908, #5794, #12525, #2068, #9124, #15822, #3618, #15723, #17043, #8798, #1955, #8685, #15408, #306, #9012, #13849, #518, #5470, #12192, #3830, #7254, #20693, #19039, #5576, #10666, #17368, #7792, #5904, #1167, #1058, #16150, #14496, #17692, #17584, #6343, #4460, #9232, #7692, #16258, #17904, #2491, #12847, #6230, #14718, #15931, #9333, #7900, #14603, #21342, #19567, #12960, #21238, #21453, #11296, #2594, #21021, #2817, #7577, #10979, #10883, #16033, #842, #9555, #12634, #8010, #11192, #16364, #9664, #19684, #19355, #6117, #19250, #14276, #18018, #4153, #12740, #4253, #9450, #4575, #2929, #17796, #11082, #1276, #946, #14388, #21128, #6011, #19463, #4353, #2705, #13508, #20242, #13400, #18248, #5134, #20134, #15159, #16696, #6693, #10212, #1385, #21786, #13069, #10098, #5028, #9993, #19796, #3149, #1498, #11852, #8228, #21564, #18128, #18471, #1604, #59, #3487, #11737, #3374, #6801, #4687, #11404, #18581, #14930, #20030, #16915, #9775, #9880, #1827, #8560, #171, #16579, #21678, #16806, #6574, #13292, #1721, #15272, #4915, #3037, #16471, #8114, #11628, #8454 ) ),
 .UNSPECIFIED., .T., .F., .F. ) 
 B_SPLINE_SURFACE_WITH_KNOTS ( ( 4, 3, 4 ),
 ( 4, 2, 2, 2, 2, 2, 2, 2, 2, 2, 2, 2, 2, 2, 2, 2, 2, 2, 2, 2, 2, 2, 2, 2, 2, 2, 2, 2, 2, 2, 2, 2, 2, 2, 2, 2, 2, 2, 2, 2, 2, 2, 2, 2, 2, 2, 2, 2, 2, 2, 2, 2, 2, 2, 2, 2, 2, 2, 2, 2, 2, 2, 2, 2, 2, 2, 2, 2, 2, 2, 2, 2, 2, 2, 2, 2, 2, 2, 2, 2, 4 ),
 ( 0.000000000000000000, 0.5000000000000000000, 1.000000000000000000 ),
 ( 0.000000000000000000, 0.008318061648474830982, 0.01871563870907547167, 0.02911321576967611582, 0.03951079283027675998, 0.04990836989087740067, 0.06030594695147804829, 0.07070352401207868898, 0.08110110107267932966, 0.09149867813327997035, 0.1018962551938805972, 0.1122938322544812378, 0.1226914093150818785, 0.1330889863756825053, 0.1434865634362831321, 0.1538841404968837590, 0.1642817175574843858, 0.1746792946180850126, 0.1850768716786856394, 0.1954744487392862939, 0.2058720257998869485, 0.2162696028604875753, 0.2266671799210882021, 0.2370647569816888289, 0.2474623340422894557, 0.2578599111028900825, 0.2682574881634907094, 0.2786550652240913362, 0.2890526422846919630, 0.2994502193452925343, 0.3098477964058931611, 0.3202453734664937879, 0.3306429505270944147, 0.3410405275876950415, 0.3514381046482956683, 0.3618356817088962951, 0.3722332587694969219, 0.3826308358300975487, 0.3930284128906983421, 0.4034259899512990799, 0.4138235670118998732, 0.4242211440725006666, 0.4346187211331002942, 0.4450162981936999218, 0.4554138752542995494, 0.4658114523148991770, 0.4762090293755006920, 0.4866066064361021515, 0.4970041834967036110, 0.5074017605573051259, 0.5177993376179057528, 0.5281969146785063796, 0.5385944917391070064, 0.5489920687997077442, 0.5593896458603083710, 0.5697872229209089978, 0.5801847999815096246, 0.5905823770421102514, 0.6009799541027108782, 0.6113775311633115050, 0.6217751082239121319, 0.6321726852845127587, 0.6425702623451133855, 0.6529678394057140123, 0.6633654164663146391, 0.6737629935269152659, 0.6841605705875142274, 0.6945581476481130778, 0.7049557247087120393, 0.7153533017693110008, 0.7257508788299132929, 0.7361484558905155851, 0.7465460329511179882, 0.7569436100117202804, 0.7673411870723210182, 0.7777387641329216450, 0.7881363411935222718, 0.7985339182541228986, 0.8080132075800156022, 0.8174924969059083057, 0.8280181261579530050 ),
 .UNSPECIFIED. ) 
 GEOMETRIC_REPRESENTATION_ITEM ( )  RATIONAL_B_SPLINE_SURFACE ( (
 ( 1.000000000000000000, 1.000000000000000000, 1.000000000000000000, 1.000000000000000000, 1.000000000000000000, 1.000000000000000000, 1.000000000000000000, 1.000000000000000000, 1.000000000000000000, 1.000000000000000000, 1.000000000000000000, 1.000000000000000000, 1.000000000000000000, 1.000000000000000000, 1.000000000000000000, 1.000000000000000000, 1.000000000000000000, 1.000000000000000000, 1.000000000000000000, 1.000000000000000000, 1.000000000000000000, 1.000000000000000000, 1.000000000000000000, 1.000000000000000000, 1.000000000000000000, 1.000000000000000000, 1.000000000000000000, 1.000000000000000000, 1.000000000000000000, 1.000000000000000000, 1.000000000000000000, 1.000000000000000000, 1.000000000000000000, 1.000000000000000000, 1.000000000000000000, 1.000000000000000000, 1.000000000000000000, 1.000000000000000000, 1.000000000000000000, 1.000000000000000000, 1.000000000000000000, 1.000000000000000000, 1.000000000000000000, 1.000000000000000000, 1.000000000000000000, 1.000000000000000000, 1.000000000000000000, 1.000000000000000000, 1.000000000000000000, 1.000000000000000000, 1.000000000000000000, 1.000000000000000000, 1.000000000000000000, 1.000000000000000000, 1.000000000000000000, 1.000000000000000000, 1.000000000000000000, 1.000000000000000000, 1.000000000000000000, 1.000000000000000000, 1.000000000000000000, 1.000000000000000000, 1.000000000000000000, 1.000000000000000000, 1.000000000000000000, 1.000000000000000000, 1.000000000000000000, 1.000000000000000000, 1.000000000000000000, 1.000000000000000000, 1.000000000000000000, 1.000000000000000000, 1.000000000000000000, 1.000000000000000000, 1.000000000000000000, 1.000000000000000000, 1.000000000000000000, 1.000000000000000000, 1.000000000000000000, 1.000000000000000000, 1.000000000000000000, 1.000000000000000000, 1.000000000000000000, 1.000000000000000000, 1.000000000000000000, 1.000000000000000000, 1.000000000000000000, 1.000000000000000000, 1.000000000000000000, 1.000000000000000000, 1.000000000000000000, 1.000000000000000000, 1.000000000000000000, 1.000000000000000000, 1.000000000000000000, 1.000000000000000000, 1.000000000000000000, 1.000000000000000000, 1.000000000000000000, 1.000000000000000000, 1.000000000000000000, 1.000000000000000000, 1.000000000000000000, 1.000000000000000000, 1.000000000000000000, 1.000000000000000000, 1.000000000000000000, 1.000000000000000000, 1.000000000000000000, 1.000000000000000000, 1.000000000000000000, 1.000000000000000000, 1.000000000000000000, 1.000000000000000000, 1.000000000000000000, 1.000000000000000000, 1.000000000000000000, 1.000000000000000000, 1.000000000000000000, 1.000000000000000000, 1.000000000000000000, 1.000000000000000000, 1.000000000000000000, 1.000000000000000000, 1.000000000000000000, 1.000000000000000000, 1.000000000000000000, 1.000000000000000000, 1.000000000000000000, 1.000000000000000000, 1.000000000000000000, 1.000000000000000000, 1.000000000000000000, 1.000000000000000000, 1.000000000000000000, 1.000000000000000000, 1.000000000000000000, 1.000000000000000000, 1.000000000000000000, 1.000000000000000000, 1.000000000000000000, 1.000000000000000000, 1.000000000000000000, 1.000000000000000000, 1.000000000000000000, 1.000000000000000000, 1.000000000000000000, 1.000000000000000000, 1.000000000000000000, 1.000000000000000000, 1.000000000000000000, 1.000000000000000000, 1.000000000000000000, 1.000000000000000000, 1.000000000000000000, 1.000000000000000000, 1.000000000000000000, 1.000000000000000000, 1.000000000000000000, 1.000000000000000000, 1.000000000000000000, 1.000000000000000000),
 ( 0.3333333333333333703, 0.3333333333333333703, 0.3333333333333333703, 0.3333333333333333703, 0.3333333333333333703, 0.3333333333333333703, 0.3333333333333333703, 0.3333333333333333703, 0.3333333333333333703, 0.3333333333333333703, 0.3333333333333333703, 0.3333333333333333703, 0.3333333333333333703, 0.3333333333333333703, 0.3333333333333333703, 0.3333333333333333703, 0.3333333333333333703, 0.3333333333333333703, 0.3333333333333333703, 0.3333333333333333703, 0.3333333333333333703, 0.3333333333333333703, 0.3333333333333333703, 0.3333333333333333703, 0.3333333333333333703, 0.3333333333333333703, 0.3333333333333333703, 0.3333333333333333703, 0.3333333333333333703, 0.3333333333333333703, 0.3333333333333333703, 0.3333333333333333703, 0.3333333333333333703, 0.3333333333333333703, 0.3333333333333333703, 0.3333333333333333703, 0.3333333333333333703, 0.3333333333333333703, 0.3333333333333333703, 0.3333333333333333703, 0.3333333333333333703, 0.3333333333333333703, 0.3333333333333333703, 0.3333333333333333703, 0.3333333333333333703, 0.3333333333333333703, 0.3333333333333333703, 0.3333333333333333703, 0.3333333333333333703, 0.3333333333333333703, 0.3333333333333333703, 0.3333333333333333703, 0.3333333333333333703, 0.3333333333333333703, 0.3333333333333333703, 0.3333333333333333703, 0.3333333333333333703, 0.3333333333333333703, 0.3333333333333333703, 0.3333333333333333703, 0.3333333333333333703, 0.3333333333333333703, 0.3333333333333333703, 0.3333333333333333703, 0.3333333333333333703, 0.3333333333333333703, 0.3333333333333333703, 0.3333333333333333703, 0.3333333333333333703, 0.3333333333333333703, 0.3333333333333333703, 0.3333333333333333703, 0.3333333333333333703, 0.3333333333333333703, 0.3333333333333333703, 0.3333333333333333703, 0.3333333333333333703, 0.3333333333333333703, 0.3333333333333333703, 0.3333333333333333703, 0.3333333333333333703, 0.3333333333333333703, 0.3333333333333333703, 0.3333333333333333703, 0.3333333333333333703, 0.3333333333333333703, 0.3333333333333333703, 0.3333333333333333703, 0.3333333333333333703, 0.3333333333333333703, 0.3333333333333333703, 0.3333333333333333703, 0.3333333333333333703, 0.3333333333333333703, 0.3333333333333333703, 0.3333333333333333703, 0.3333333333333333703, 0.3333333333333333703, 0.3333333333333333703, 0.3333333333333333703, 0.3333333333333333703, 0.3333333333333333703, 0.3333333333333333703, 0.3333333333333333703, 0.3333333333333333703, 0.3333333333333333703, 0.3333333333333333703, 0.3333333333333333703, 0.3333333333333333703, 0.3333333333333333703, 0.3333333333333333703, 0.3333333333333333703, 0.3333333333333333703, 0.3333333333333333703, 0.3333333333333333703, 0.3333333333333333703, 0.3333333333333333703, 0.3333333333333333703, 0.3333333333333333703, 0.3333333333333333703, 0.3333333333333333703, 0.3333333333333333703, 0.3333333333333333703, 0.3333333333333333703, 0.3333333333333333703, 0.3333333333333333703, 0.3333333333333333703, 0.3333333333333333703, 0.3333333333333333703, 0.3333333333333333703, 0.3333333333333333703, 0.3333333333333333703, 0.3333333333333333703, 0.3333333333333333703, 0.3333333333333333703, 0.3333333333333333703, 0.3333333333333333703, 0.3333333333333333703, 0.3333333333333333703, 0.3333333333333333703, 0.3333333333333333703, 0.3333333333333333703, 0.3333333333333333703, 0.3333333333333333703, 0.3333333333333333703, 0.3333333333333333703, 0.3333333333333333703, 0.3333333333333333703, 0.3333333333333333703, 0.3333333333333333703, 0.3333333333333333703, 0.3333333333333333703, 0.3333333333333333703, 0.3333333333333333703, 0.3333333333333333703, 0.3333333333333333703, 0.3333333333333333703, 0.3333333333333333703, 0.3333333333333333703, 0.3333333333333333703, 0.3333333333333333703, 0.3333333333333333703),
 ( 0.3333333333333333703, 0.3333333333333333703, 0.3333333333333333703, 0.3333333333333333703, 0.3333333333333333703, 0.3333333333333333703, 0.3333333333333333703, 0.3333333333333333703, 0.3333333333333333703, 0.3333333333333333703, 0.3333333333333333703, 0.3333333333333333703, 0.3333333333333333703, 0.3333333333333333703, 0.3333333333333333703, 0.3333333333333333703, 0.3333333333333333703, 0.3333333333333333703, 0.3333333333333333703, 0.3333333333333333703, 0.3333333333333333703, 0.3333333333333333703, 0.3333333333333333703, 0.3333333333333333703, 0.3333333333333333703, 0.3333333333333333703, 0.3333333333333333703, 0.3333333333333333703, 0.3333333333333333703, 0.3333333333333333703, 0.3333333333333333703, 0.3333333333333333703, 0.3333333333333333703, 0.3333333333333333703, 0.3333333333333333703, 0.3333333333333333703, 0.3333333333333333703, 0.3333333333333333703, 0.3333333333333333703, 0.3333333333333333703, 0.3333333333333333703, 0.3333333333333333703, 0.3333333333333333703, 0.3333333333333333703, 0.3333333333333333703, 0.3333333333333333703, 0.3333333333333333703, 0.3333333333333333703, 0.3333333333333333703, 0.3333333333333333703, 0.3333333333333333703, 0.3333333333333333703, 0.3333333333333333703, 0.3333333333333333703, 0.3333333333333333703, 0.3333333333333333703, 0.3333333333333333703, 0.3333333333333333703, 0.3333333333333333703, 0.3333333333333333703, 0.3333333333333333703, 0.3333333333333333703, 0.3333333333333333703, 0.3333333333333333703, 0.3333333333333333703, 0.3333333333333333703, 0.3333333333333333703, 0.3333333333333333703, 0.3333333333333333703, 0.3333333333333333703, 0.3333333333333333703, 0.3333333333333333703, 0.3333333333333333703, 0.3333333333333333703, 0.3333333333333333703, 0.3333333333333333703, 0.3333333333333333703, 0.3333333333333333703, 0.3333333333333333703, 0.3333333333333333703, 0.3333333333333333703, 0.3333333333333333703, 0.3333333333333333703, 0.3333333333333333703, 0.3333333333333333703, 0.3333333333333333703, 0.3333333333333333703, 0.3333333333333333703, 0.3333333333333333703, 0.3333333333333333703, 0.3333333333333333703, 0.3333333333333333703, 0.3333333333333333703, 0.3333333333333333703, 0.3333333333333333703, 0.3333333333333333703, 0.3333333333333333703, 0.3333333333333333703, 0.3333333333333333703, 0.3333333333333333703, 0.3333333333333333703, 0.3333333333333333703, 0.3333333333333333703, 0.3333333333333333703, 0.3333333333333333703, 0.3333333333333333703, 0.3333333333333333703, 0.3333333333333333703, 0.3333333333333333703, 0.3333333333333333703, 0.3333333333333333703, 0.3333333333333333703, 0.3333333333333333703, 0.3333333333333333703, 0.3333333333333333703, 0.3333333333333333703, 0.3333333333333333703, 0.3333333333333333703, 0.3333333333333333703, 0.3333333333333333703, 0.3333333333333333703, 0.3333333333333333703, 0.3333333333333333703, 0.3333333333333333703, 0.3333333333333333703, 0.3333333333333333703, 0.3333333333333333703, 0.3333333333333333703, 0.3333333333333333703, 0.3333333333333333703, 0.3333333333333333703, 0.3333333333333333703, 0.3333333333333333703, 0.3333333333333333703, 0.3333333333333333703, 0.3333333333333333703, 0.3333333333333333703, 0.3333333333333333703, 0.3333333333333333703, 0.3333333333333333703, 0.3333333333333333703, 0.3333333333333333703, 0.3333333333333333703, 0.3333333333333333703, 0.3333333333333333703, 0.3333333333333333703, 0.3333333333333333703, 0.3333333333333333703, 0.3333333333333333703, 0.3333333333333333703, 0.3333333333333333703, 0.3333333333333333703, 0.3333333333333333703, 0.3333333333333333703, 0.3333333333333333703, 0.3333333333333333703, 0.3333333333333333703, 0.3333333333333333703, 0.3333333333333333703, 0.3333333333333333703, 0.3333333333333333703, 0.3333333333333333703),
 ( 1.000000000000000000, 1.000000000000000000, 1.000000000000000000, 1.000000000000000000, 1.000000000000000000, 1.000000000000000000, 1.000000000000000000, 1.000000000000000000, 1.000000000000000000, 1.000000000000000000, 1.000000000000000000, 1.000000000000000000, 1.000000000000000000, 1.000000000000000000, 1.000000000000000000, 1.000000000000000000, 1.000000000000000000, 1.000000000000000000, 1.000000000000000000, 1.000000000000000000, 1.000000000000000000, 1.000000000000000000, 1.000000000000000000, 1.000000000000000000, 1.000000000000000000, 1.000000000000000000, 1.000000000000000000, 1.000000000000000000, 1.000000000000000000, 1.000000000000000000, 1.000000000000000000, 1.000000000000000000, 1.000000000000000000, 1.000000000000000000, 1.000000000000000000, 1.000000000000000000, 1.000000000000000000, 1.000000000000000000, 1.000000000000000000, 1.000000000000000000, 1.000000000000000000, 1.000000000000000000, 1.000000000000000000, 1.000000000000000000, 1.000000000000000000, 1.000000000000000000, 1.000000000000000000, 1.000000000000000000, 1.000000000000000000, 1.000000000000000000, 1.000000000000000000, 1.000000000000000000, 1.000000000000000000, 1.000000000000000000, 1.000000000000000000, 1.000000000000000000, 1.000000000000000000, 1.000000000000000000, 1.000000000000000000, 1.000000000000000000, 1.000000000000000000, 1.000000000000000000, 1.000000000000000000, 1.000000000000000000, 1.000000000000000000, 1.000000000000000000, 1.000000000000000000, 1.000000000000000000, 1.000000000000000000, 1.000000000000000000, 1.000000000000000000, 1.000000000000000000, 1.000000000000000000, 1.000000000000000000, 1.000000000000000000, 1.000000000000000000, 1.000000000000000000, 1.000000000000000000, 1.000000000000000000, 1.000000000000000000, 1.000000000000000000, 1.000000000000000000, 1.000000000000000000, 1.000000000000000000, 1.000000000000000000, 1.000000000000000000, 1.000000000000000000, 1.000000000000000000, 1.000000000000000000, 1.000000000000000000, 1.000000000000000000, 1.000000000000000000, 1.000000000000000000, 1.000000000000000000, 1.000000000000000000, 1.000000000000000000, 1.000000000000000000, 1.000000000000000000, 1.000000000000000000, 1.000000000000000000, 1.000000000000000000, 1.000000000000000000, 1.000000000000000000, 1.000000000000000000, 1.000000000000000000, 1.000000000000000000, 1.000000000000000000, 1.000000000000000000, 1.000000000000000000, 1.000000000000000000, 1.000000000000000000, 1.000000000000000000, 1.000000000000000000, 1.000000000000000000, 1.000000000000000000, 1.000000000000000000, 1.000000000000000000, 1.000000000000000000, 1.000000000000000000, 1.000000000000000000, 1.000000000000000000, 1.000000000000000000, 1.000000000000000000, 1.000000000000000000, 1.000000000000000000, 1.000000000000000000, 1.000000000000000000, 1.000000000000000000, 1.000000000000000000, 1.000000000000000000, 1.000000000000000000, 1.000000000000000000, 1.000000000000000000, 1.000000000000000000, 1.000000000000000000, 1.000000000000000000, 1.000000000000000000, 1.000000000000000000, 1.000000000000000000, 1.000000000000000000, 1.000000000000000000, 1.000000000000000000, 1.000000000000000000, 1.000000000000000000, 1.000000000000000000, 1.000000000000000000, 1.000000000000000000, 1.000000000000000000, 1.000000000000000000, 1.000000000000000000, 1.000000000000000000, 1.000000000000000000, 1.000000000000000000, 1.000000000000000000, 1.000000000000000000, 1.000000000000000000, 1.000000000000000000, 1.000000000000000000, 1.000000000000000000, 1.000000000000000000, 1.000000000000000000, 1.000000000000000000),
 ( 0.3333333333333333703, 0.3333333333333333703, 0.3333333333333333703, 0.3333333333333333703, 0.3333333333333333703, 0.3333333333333333703, 0.3333333333333333703, 0.3333333333333333703, 0.3333333333333333703, 0.3333333333333333703, 0.3333333333333333703, 0.3333333333333333703, 0.3333333333333333703, 0.3333333333333333703, 0.3333333333333333703, 0.3333333333333333703, 0.3333333333333333703, 0.3333333333333333703, 0.3333333333333333703, 0.3333333333333333703, 0.3333333333333333703, 0.3333333333333333703, 0.3333333333333333703, 0.3333333333333333703, 0.3333333333333333703, 0.3333333333333333703, 0.3333333333333333703, 0.3333333333333333703, 0.3333333333333333703, 0.3333333333333333703, 0.3333333333333333703, 0.3333333333333333703, 0.3333333333333333703, 0.3333333333333333703, 0.3333333333333333703, 0.3333333333333333703, 0.3333333333333333703, 0.3333333333333333703, 0.3333333333333333703, 0.3333333333333333703, 0.3333333333333333703, 0.3333333333333333703, 0.3333333333333333703, 0.3333333333333333703, 0.3333333333333333703, 0.3333333333333333703, 0.3333333333333333703, 0.3333333333333333703, 0.3333333333333333703, 0.3333333333333333703, 0.3333333333333333703, 0.3333333333333333703, 0.3333333333333333703, 0.3333333333333333703, 0.3333333333333333703, 0.3333333333333333703, 0.3333333333333333703, 0.3333333333333333703, 0.3333333333333333703, 0.3333333333333333703, 0.3333333333333333703, 0.3333333333333333703, 0.3333333333333333703, 0.3333333333333333703, 0.3333333333333333703, 0.3333333333333333703, 0.3333333333333333703, 0.3333333333333333703, 0.3333333333333333703, 0.3333333333333333703, 0.3333333333333333703, 0.3333333333333333703, 0.3333333333333333703, 0.3333333333333333703, 0.3333333333333333703, 0.3333333333333333703, 0.3333333333333333703, 0.3333333333333333703, 0.3333333333333333703, 0.3333333333333333703, 0.3333333333333333703, 0.3333333333333333703, 0.3333333333333333703, 0.3333333333333333703, 0.3333333333333333703, 0.3333333333333333703, 0.3333333333333333703, 0.3333333333333333703, 0.3333333333333333703, 0.3333333333333333703, 0.3333333333333333703, 0.3333333333333333703, 0.3333333333333333703, 0.3333333333333333703, 0.3333333333333333703, 0.3333333333333333703, 0.3333333333333333703, 0.3333333333333333703, 0.3333333333333333703, 0.3333333333333333703, 0.3333333333333333703, 0.3333333333333333703, 0.3333333333333333703, 0.3333333333333333703, 0.3333333333333333703, 0.3333333333333333703, 0.3333333333333333703, 0.3333333333333333703, 0.3333333333333333703, 0.3333333333333333703, 0.3333333333333333703, 0.3333333333333333703, 0.3333333333333333703, 0.3333333333333333703, 0.3333333333333333703, 0.3333333333333333703, 0.3333333333333333703, 0.3333333333333333703, 0.3333333333333333703, 0.3333333333333333703, 0.3333333333333333703, 0.3333333333333333703, 0.3333333333333333703, 0.3333333333333333703, 0.3333333333333333703, 0.3333333333333333703, 0.3333333333333333703, 0.3333333333333333703, 0.3333333333333333703, 0.3333333333333333703, 0.3333333333333333703, 0.3333333333333333703, 0.3333333333333333703, 0.3333333333333333703, 0.3333333333333333703, 0.3333333333333333703, 0.3333333333333333703, 0.3333333333333333703, 0.3333333333333333703, 0.3333333333333333703, 0.3333333333333333703, 0.3333333333333333703, 0.3333333333333333703, 0.3333333333333333703, 0.3333333333333333703, 0.3333333333333333703, 0.3333333333333333703, 0.3333333333333333703, 0.3333333333333333703, 0.3333333333333333703, 0.3333333333333333703, 0.3333333333333333703, 0.3333333333333333703, 0.3333333333333333703, 0.3333333333333333703, 0.3333333333333333703, 0.3333333333333333703, 0.3333333333333333703, 0.3333333333333333703, 0.3333333333333333703, 0.3333333333333333703, 0.3333333333333333703),
 ( 0.3333333333333333703, 0.3333333333333333703, 0.3333333333333333703, 0.3333333333333333703, 0.3333333333333333703, 0.3333333333333333703, 0.3333333333333333703, 0.3333333333333333703, 0.3333333333333333703, 0.3333333333333333703, 0.3333333333333333703, 0.3333333333333333703, 0.3333333333333333703, 0.3333333333333333703, 0.3333333333333333703, 0.3333333333333333703, 0.3333333333333333703, 0.3333333333333333703, 0.3333333333333333703, 0.3333333333333333703, 0.3333333333333333703, 0.3333333333333333703, 0.3333333333333333703, 0.3333333333333333703, 0.3333333333333333703, 0.3333333333333333703, 0.3333333333333333703, 0.3333333333333333703, 0.3333333333333333703, 0.3333333333333333703, 0.3333333333333333703, 0.3333333333333333703, 0.3333333333333333703, 0.3333333333333333703, 0.3333333333333333703, 0.3333333333333333703, 0.3333333333333333703, 0.3333333333333333703, 0.3333333333333333703, 0.3333333333333333703, 0.3333333333333333703, 0.3333333333333333703, 0.3333333333333333703, 0.3333333333333333703, 0.3333333333333333703, 0.3333333333333333703, 0.3333333333333333703, 0.3333333333333333703, 0.3333333333333333703, 0.3333333333333333703, 0.3333333333333333703, 0.3333333333333333703, 0.3333333333333333703, 0.3333333333333333703, 0.3333333333333333703, 0.3333333333333333703, 0.3333333333333333703, 0.3333333333333333703, 0.3333333333333333703, 0.3333333333333333703, 0.3333333333333333703, 0.3333333333333333703, 0.3333333333333333703, 0.3333333333333333703, 0.3333333333333333703, 0.3333333333333333703, 0.3333333333333333703, 0.3333333333333333703, 0.3333333333333333703, 0.3333333333333333703, 0.3333333333333333703, 0.3333333333333333703, 0.3333333333333333703, 0.3333333333333333703, 0.3333333333333333703, 0.3333333333333333703, 0.3333333333333333703, 0.3333333333333333703, 0.3333333333333333703, 0.3333333333333333703, 0.3333333333333333703, 0.3333333333333333703, 0.3333333333333333703, 0.3333333333333333703, 0.3333333333333333703, 0.3333333333333333703, 0.3333333333333333703, 0.3333333333333333703, 0.3333333333333333703, 0.3333333333333333703, 0.3333333333333333703, 0.3333333333333333703, 0.3333333333333333703, 0.3333333333333333703, 0.3333333333333333703, 0.3333333333333333703, 0.3333333333333333703, 0.3333333333333333703, 0.3333333333333333703, 0.3333333333333333703, 0.3333333333333333703, 0.3333333333333333703, 0.3333333333333333703, 0.3333333333333333703, 0.3333333333333333703, 0.3333333333333333703, 0.3333333333333333703, 0.3333333333333333703, 0.3333333333333333703, 0.3333333333333333703, 0.3333333333333333703, 0.3333333333333333703, 0.3333333333333333703, 0.3333333333333333703, 0.3333333333333333703, 0.3333333333333333703, 0.3333333333333333703, 0.3333333333333333703, 0.3333333333333333703, 0.3333333333333333703, 0.3333333333333333703, 0.3333333333333333703, 0.3333333333333333703, 0.3333333333333333703, 0.3333333333333333703, 0.3333333333333333703, 0.3333333333333333703, 0.3333333333333333703, 0.3333333333333333703, 0.3333333333333333703, 0.3333333333333333703, 0.3333333333333333703, 0.3333333333333333703, 0.3333333333333333703, 0.3333333333333333703, 0.3333333333333333703, 0.3333333333333333703, 0.3333333333333333703, 0.3333333333333333703, 0.3333333333333333703, 0.3333333333333333703, 0.3333333333333333703, 0.3333333333333333703, 0.3333333333333333703, 0.3333333333333333703, 0.3333333333333333703, 0.3333333333333333703, 0.3333333333333333703, 0.3333333333333333703, 0.3333333333333333703, 0.3333333333333333703, 0.3333333333333333703, 0.3333333333333333703, 0.3333333333333333703, 0.3333333333333333703, 0.3333333333333333703, 0.3333333333333333703, 0.3333333333333333703, 0.3333333333333333703, 0.3333333333333333703, 0.3333333333333333703, 0.3333333333333333703),
 ( 1.000000000000000000, 1.000000000000000000, 1.000000000000000000, 1.000000000000000000, 1.000000000000000000, 1.000000000000000000, 1.000000000000000000, 1.000000000000000000, 1.000000000000000000, 1.000000000000000000, 1.000000000000000000, 1.000000000000000000, 1.000000000000000000, 1.000000000000000000, 1.000000000000000000, 1.000000000000000000, 1.000000000000000000, 1.000000000000000000, 1.000000000000000000, 1.000000000000000000, 1.000000000000000000, 1.000000000000000000, 1.000000000000000000, 1.000000000000000000, 1.000000000000000000, 1.000000000000000000, 1.000000000000000000, 1.000000000000000000, 1.000000000000000000, 1.000000000000000000, 1.000000000000000000, 1.000000000000000000, 1.000000000000000000, 1.000000000000000000, 1.000000000000000000, 1.000000000000000000, 1.000000000000000000, 1.000000000000000000, 1.000000000000000000, 1.000000000000000000, 1.000000000000000000, 1.000000000000000000, 1.000000000000000000, 1.000000000000000000, 1.000000000000000000, 1.000000000000000000, 1.000000000000000000, 1.000000000000000000, 1.000000000000000000, 1.000000000000000000, 1.000000000000000000, 1.000000000000000000, 1.000000000000000000, 1.000000000000000000, 1.000000000000000000, 1.000000000000000000, 1.000000000000000000, 1.000000000000000000, 1.000000000000000000, 1.000000000000000000, 1.000000000000000000, 1.000000000000000000, 1.000000000000000000, 1.000000000000000000, 1.000000000000000000, 1.000000000000000000, 1.000000000000000000, 1.000000000000000000, 1.000000000000000000, 1.000000000000000000, 1.000000000000000000, 1.000000000000000000, 1.000000000000000000, 1.000000000000000000, 1.000000000000000000, 1.000000000000000000, 1.000000000000000000, 1.000000000000000000, 1.000000000000000000, 1.000000000000000000, 1.000000000000000000, 1.000000000000000000, 1.000000000000000000, 1.000000000000000000, 1.000000000000000000, 1.000000000000000000, 1.000000000000000000, 1.000000000000000000, 1.000000000000000000, 1.000000000000000000, 1.000000000000000000, 1.000000000000000000, 1.000000000000000000, 1.000000000000000000, 1.000000000000000000, 1.000000000000000000, 1.000000000000000000, 1.000000000000000000, 1.000000000000000000, 1.000000000000000000, 1.000000000000000000, 1.000000000000000000, 1.000000000000000000, 1.000000000000000000, 1.000000000000000000, 1.000000000000000000, 1.000000000000000000, 1.000000000000000000, 1.000000000000000000, 1.000000000000000000, 1.000000000000000000, 1.000000000000000000, 1.000000000000000000, 1.000000000000000000, 1.000000000000000000, 1.000000000000000000, 1.000000000000000000, 1.000000000000000000, 1.000000000000000000, 1.000000000000000000, 1.000000000000000000, 1.000000000000000000, 1.000000000000000000, 1.000000000000000000, 1.000000000000000000, 1.000000000000000000, 1.000000000000000000, 1.000000000000000000, 1.000000000000000000, 1.000000000000000000, 1.000000000000000000, 1.000000000000000000, 1.000000000000000000, 1.000000000000000000, 1.000000000000000000, 1.000000000000000000, 1.000000000000000000, 1.000000000000000000, 1.000000000000000000, 1.000000000000000000, 1.000000000000000000, 1.000000000000000000, 1.000000000000000000, 1.000000000000000000, 1.000000000000000000, 1.000000000000000000, 1.000000000000000000, 1.000000000000000000, 1.000000000000000000, 1.000000000000000000, 1.000000000000000000, 1.000000000000000000, 1.000000000000000000, 1.000000000000000000, 1.000000000000000000, 1.000000000000000000, 1.000000000000000000, 1.000000000000000000, 1.000000000000000000, 1.000000000000000000, 1.000000000000000000, 1.000000000000000000) ) ) 
 REPRESENTATION_ITEM ( '' )  SURFACE ( )  );
#14596=CARTESIAN_POINT ( 'NONE',  ( 43.06284635655732274, 148.1064719378950088, -10.08176808973812655 ) ) ;
#14603=CARTESIAN_POINT ( 'NONE',  ( 40.02721236285810136, 85.80382532021769748, 0.4343372985580923329 ) ) ;
#14604=CARTESIAN_POINT ( 'NONE',  ( 22.52008984372607614, 139.2495111981779985, 17.01435058386764965 ) ) ;
#14622=CARTESIAN_POINT ( 'NONE',  ( 43.13803657676253067, 85.59359249887060628, 13.33475322466254198 ) ) ;
#14626=CARTESIAN_POINT ( 'NONE',  ( 68.01140435219951996, 119.9070776186055838, 50.00000000000002842 ) ) ;
#14628=CARTESIAN_POINT ( 'NONE',  ( 70.35668680342836012, 113.0167181193761508, -8.057780719902234878 ) ) ;
#14632=SHAPE_REPRESENTATION ( 'Handle Balance Tension Spring', ( #12657 ), #19020 ) ;
#14639=CARTESIAN_POINT ( 'NONE',  ( 39.14927582833848874, 92.05416703502255871, 8.565614722876343734 ) ) ;
#14658=CARTESIAN_POINT ( 'NONE',  ( 14.54084317601859588, 100.7536435603138756, 21.43002817983359876 ) ) ;
#14660=CARTESIAN_POINT ( 'NONE',  ( 9.046145050308979307, 123.4917717844193277, -10.79923121120670437 ) ) ;
#14665=CARTESIAN_POINT ( 'NONE',  ( 20.99626426110969390, 137.5292218135913913, 9.918250401459649979 ) ) ;
#14671=CARTESIAN_POINT ( 'NONE',  ( 15.96294818963569639, 111.9339314265907745, 8.846935114401974332 ) ) ;
#14673=CARTESIAN_POINT ( 'NONE',  ( 76.66991938639012005, 113.6622739410785670, 5.791450954060403333 ) ) ;
#14684=CARTESIAN_POINT ( 'NONE',  ( 57.78275410301085913, 89.02518083909171764, -0.1607367497116551913 ) ) ;
#14690=VECTOR ( 'NONE', #781, 1000.000000000000114 ) ;
#14705=CARTESIAN_POINT ( 'NONE',  ( 53.01140435219953417, 119.9070776186055838, -19.99999999999998579 ) ) ;
#14711=CARTESIAN_POINT ( 'NONE',  ( 16.54882264740998110, 129.8072851447780067, 22.56993813403257931 ) ) ;
#14715=ORIENTED_EDGE ( 'NONE', *, *, #7470, .F. ) ;
#14718=CARTESIAN_POINT ( 'NONE',  ( 61.01612483116806374, 90.79174121657607088, -0.2798613066081144796 ) ) ;
#14719=CARTESIAN_POINT ( 'NONE',  ( 60.58642193167724344, 97.95666160567475345, -13.33918631239395225 ) ) ;
#14733=( LENGTH_UNIT ( ) NAMED_UNIT ( * ) SI_UNIT ( .MILLI., .METRE. ) );
#14736=CARTESIAN_POINT ( 'NONE',  ( 30.67228459367742133, 151.9265198579663263, 16.42994147312239051 ) ) ;
#14743=CARTESIAN_POINT ( 'NONE',  ( 67.11143925497957241, 134.7062941969633414, 18.05698923925237764 ) ) ;
#14751=CARTESIAN_POINT ( 'NONE',  ( 70.48507635059884535, 125.9029633330538189, 6.422671151982867421 ) ) ;
#14761=CARTESIAN_POINT ( 'NONE',  ( 42.92180000979148957, 85.67454126555050209, 7.339147150375312734 ) ) ;
#14769=CARTESIAN_POINT ( 'NONE',  ( 75.73800832010900308, 109.5907576069244698, 18.92991194937467014 ) ) ;
#14772=CARTESIAN_POINT ( 'NONE',  ( 50.69626032627856915, 86.62977272806217854, -5.918438612465169335 ) ) ;
#14776=CARTESIAN_POINT ( 'NONE',  ( 17.98614708603287937, 106.9092867359673704, 15.63253669370310384 ) ) ;
#14781=CARTESIAN_POINT ( 'NONE',  ( 24.77189431714078083, 141.4131305960171687, 3.132649400142189844 ) ) ;
#14793=CARTESIAN_POINT ( 'NONE',  ( 34.41316853928974950, 153.0433231119815503, 10.55326060710041958 ) ) ;
#14803=STYLED_ITEM ( 'NONE', ( #334 ), #353 ) ;
#14814=CARTESIAN_POINT ( 'NONE',  ( 19.91114674846567922, 103.5922903064164302, 14.48528786281536895 ) ) ;
#14821=CARTESIAN_POINT ( 'NONE',  ( 68.32201692705490359, 132.1587870917933003, -0.8393580998851425390 ) ) ;
#14837=CARTESIAN_POINT ( 'NONE',  ( 70.19659433329162823, 140.8466096914638399, 17.85851290171837746 ) ) ;
#14844=CARTESIAN_POINT ( 'NONE',  ( 10.18435502709129103, 110.4832086711448227, 2.772112504659519416 ) ) ;
#14845=CARTESIAN_POINT ( 'NONE',  ( 23.45520590541277883, 99.47716203340817742, 21.27102736060455257 ) ) ;
#14857=CARTESIAN_POINT ( 'NONE',  ( 17.95776995827587896, 107.1383635228311846, 9.636927859708212196 ) ) ;
#14864=LINE ( 'NONE', #16408, #15284 ) ;
#14869=CARTESIAN_POINT ( 'NONE',  ( 58.57487293839693621, 150.3975950434478648, 4.362879525569486994 ) ) ;
#14876=CARTESIAN_POINT ( 'NONE',  ( 62.21295035458982881, 148.3457431455455549, 17.50134052088148096 ) ) ;
#14879=CARTESIAN_POINT ( 'NONE',  ( 33.37504612857446773, 87.14074678364892179, -12.34672919366563981 ) ) ;
#14888=CARTESIAN_POINT ( 'NONE',  ( 14.93692188586762803, 117.2531131035273546, 2.061388125607503952 ) ) ;
#14899=CARTESIAN_POINT ( 'NONE',  ( 37.24990543953586553, 153.6521207556136517, 3.648881909465930828 ) ) ;
#14905=CARTESIAN_POINT ( 'NONE',  ( 64.11693453485118255, 146.8606268255622638, -2.422805558527139080 ) ) ;
#14912=CARTESIAN_POINT ( 'NONE',  ( 12.59043673732666946, 104.3826120832696773, 9.557940159192295226 ) ) ;
#14923=CARTESIAN_POINT ( 'NONE',  ( 32.78705717043479240, 146.2756902729748560, 16.50925200294354056 ) ) ;
#14929=CIRCLE ( 'NONE', #15304, 3.000000000000050626 ) ;
#14930=CARTESIAN_POINT ( 'NONE',  ( 53.04203944364535772, 87.17698241397053494, 14.00585298808814194 ) ) ;
#14932=CARTESIAN_POINT ( 'NONE',  ( 46.34060549886174840, 91.98545359010019240, -5.720099531362743406 ) ) ;
#14936=ADVANCED_FACE ( 'NONE', ( #15640 ), #1091, .T. ) ;
#14948=CARTESIAN_POINT ( 'NONE',  ( 75.41016232129729246, 131.2110917358880045, 18.21592158385217886 ) ) ;
#14953=CARTESIAN_POINT ( 'NONE',  ( 76.87285023715404009, 124.3600315475450486, -0.5611826874715375446 ) ) ;
#14954=CARTESIAN_POINT ( 'NONE',  ( 14.94677925004173957, 122.6663546818147381, -4.724578312614759135 ) ) ;
#14964=CARTESIAN_POINT ( 'NONE',  ( 59.61500273516548276, 97.21183980732109831, 0.7083854377657419210 ) ) ;
#14971=CARTESIAN_POINT ( 'NONE',  ( 68.01140435219951996, 119.9070776186055838, -19.99999999999997868 ) ) ;
#14975=CARTESIAN_POINT ( 'NONE',  ( 18.20936163119166196, 143.5026679720446907, 2.934308097026923967 ) ) ;
#14983=CARTESIAN_POINT ( 'NONE',  ( 70.07576047146775977, 128.1116393178318731, -2.657569147260473663 ) ) ;
#14986=CARTESIAN_POINT ( 'NONE',  ( 44.01981256007524479, 154.0451711359460774, -9.132611258894215212 ) ) ;
#14998=CARTESIAN_POINT ( 'NONE',  ( 28.62772086389876947, 95.65184626908498444, 8.013395860235284829 ) ) ;
#15012=CARTESIAN_POINT ( 'NONE',  ( 14.88286428391304561, 100.3963227437532595, 8.410691821786379307 ) ) ;
#15020=CARTESIAN_POINT ( 'NONE',  ( 20.91437931538276374, 145.9617080342048894, -10.94665030085253044 ) ) ;
#15023=CARTESIAN_POINT ( 'NONE',  ( 40.03295031927941494, 147.9482203214073479, -10.20071078494585670 ) ) ;
#15030=CARTESIAN_POINT ( 'NONE',  ( 27.91901995959459271, 89.26896823883201648, 8.843372880480211862 ) ) ;
#15039=CARTESIAN_POINT ( 'NONE',  ( 23.45520590541277883, 99.47716203340817742, 21.27102736060455257 ) ) ;
#15049=CARTESIAN_POINT ( 'NONE',  ( 16.96697132366095673, 109.3049078165896901, 2.732358569689224748 ) ) ;
#15066=CARTESIAN_POINT ( 'NONE',  ( 30.01547214559559507, 151.6658481390280144, 9.406004577920295873 ) ) ;
#15072=CARTESIAN_POINT ( 'NONE',  ( 76.37589548207274959, 127.2077353526990748, 6.343625931721379452 ) ) ;
#15073=CARTESIAN_POINT ( 'NONE',  ( 37.67147452025017174, 147.5968219552084122, -3.296006884014541782 ) ) ;
#15084=CARTESIAN_POINT ( 'NONE',  ( 59.05508021657500706, 143.0007772151335814, 5.589501426708507026 ) ) ;
#15094=CARTESIAN_POINT ( 'NONE',  ( 22.46358530849972723, 92.52609567587644790, 8.053519324161520387 ) ) ;
#15101=CARTESIAN_POINT ( 'NONE',  ( 70.90273821555796019, 124.5833669296562931, 4.485287862780372947 ) ) ;
#15114=CARTESIAN_POINT ( 'NONE',  ( 58.43892221570314405, 143.5117748958429047, 4.561220828673259398 ) ) ;
#15127=CARTESIAN_POINT ( 'NONE',  ( 77.21761637129371536, 122.6259224659223861, -2.498659462202352799 ) ) ;
#15134=CARTESIAN_POINT ( 'NONE',  ( 43.10205244623161036, 154.1398065127551149, -10.16071067355346358 ) ) ;
#15136=CARTESIAN_POINT ( 'NONE',  ( 37.67147452025017174, 147.5968219552084122, -3.296006884014541782 ) ) ;
#15141=CARTESIAN_POINT ( 'NONE',  ( 39.42188022582085694, 153.9507182763122159, -10.27990332573616961 ) ) ;
#15152=CARTESIAN_POINT ( 'NONE',  ( 70.35668680342836012, 113.0167181193761508, -8.057780719902234878 ) ) ;
#15159=CARTESIAN_POINT ( 'NONE',  ( 8.798315742295939046, 121.0924013121165075, 9.124689178586496752 ) ) ;
#15161=CARTESIAN_POINT ( 'NONE',  ( 15.65696388169908104, 126.4253507882334588, -3.577328847893908925 ) ) ;
#15172=B_SPLINE_CURVE_WITH_KNOTS ( 'NONE', 3,
 ( #2216, #17088, #18972, #13679, #2002, #20522, #2318, #12347, #14001, #8733, #13891, #20735, #15552, #20413, #3875, #12127, #351, #235, #18860, #15451, #7301, #556, #3984, #15766, #7186, #11920, #3767, #20629, #7081, #13783, #10709, #7406, #5309, #17412, #10494, #5511 ),
 .UNSPECIFIED., .F., .F.,
 ( 4, 2, 2, 2, 2, 2, 2, 2, 2, 2, 2, 2, 2, 2, 2, 2, 2, 4 ),
 ( 6.938893903907227607E-18, 0.0009794911224654321950, 0.001958982244930857451, 0.002938473367396282274, 0.003917964489861707963, 0.004897455612327133653, 0.005876946734792557608, 0.006856437857257983298, 0.007835928979723408988, 0.008815420102188832943, 0.009794911224654260368, 0.01028465678588698189, 0.01077440234711970514, 0.01175389346958513430, 0.01273338459205056693, 0.01371287571451599609, 0.01469236683698142872, 0.01567185795944685614 ),
 .UNSPECIFIED. ) ;
#15179=CARTESIAN_POINT ( 'NONE',  ( 10.92950091243491251, 131.9893946842779542, 22.49106082041198107 ) ) ;
#15185=CARTESIAN_POINT ( 'NONE',  ( 8.933461960486459574, 117.6319094064757422, 3.010161695468211551 ) ) ;
#15186=CARTESIAN_POINT ( 'NONE',  ( 18.92353847440636727, 134.5693106245527702, 2.775393258647981920 ) ) ;
#15198=CARTESIAN_POINT ( 'NONE',  ( 50.52618006956270591, 153.2232370340747138, -15.91843667049845834 ) ) ;
#15209=CARTESIAN_POINT ( 'NONE',  ( 13.33420504782278293, 102.8437529505761603, 1.505736668420971869 ) ) ;
#15217=CARTESIAN_POINT ( 'NONE',  ( 23.20524185134216921, 147.9029287973646660, 23.16022673208204807 ) ) ;
#15230=CARTESIAN_POINT ( 'NONE',  ( 40.25662930883660806, 147.8909896968035014, -16.19631701608006580 ) ) ;
#15237=CARTESIAN_POINT ( 'NONE',  ( 43.01140435219951996, 144.9070776186055696, 29.21067981925357060 ) ) ;
#15242=CARTESIAN_POINT ( 'NONE',  ( 51.83766784316492249, 86.74794057323931895, -0.9509610611041249273 ) ) ;
#15244=ORIENTED_EDGE ( 'NONE', *, *, #17566, .F. ) ;
#15248=CARTESIAN_POINT ( 'NONE',  ( 77.19215121279506775, 118.0176990621192203, -1.351406188750652992 ) ) ;
#15250=CARTESIAN_POINT ( 'NONE',  ( 51.94691807752363388, 146.6530262932614050, -9.724486432582017059 ) ) ;
#15255=CARTESIAN_POINT ( 'NONE',  ( 31.29766364123476663, 87.82482650329993135, 8.724447585906515812 ) ) ;
#15266=CARTESIAN_POINT ( 'NONE',  ( 66.79315400704923888, 104.7533658121278819, -7.700889860664787534 ) ) ;
#15272=CARTESIAN_POINT ( 'NONE',  ( 11.08170843061617816, 132.1625483722078513, 16.49545033792581350 ) ) ;
#15273=CARTESIAN_POINT ( 'NONE',  ( 19.10471955674299238, 134.7123306330852870, -3.220215631267630219 ) ) ;
#15284=VECTOR ( 'NONE', #6735, 1000.000000000000114 ) ;
#15292=CARTESIAN_POINT ( 'NONE',  ( 9.116869730174032682, 125.2576736736073428, 22.26325814793822744 ) ) ;
#15296=CARTESIAN_POINT ( 'NONE',  ( 17.06177112331949886, 97.70250936324737268, 2.295960169688653352 ) ) ;
#15297=CARTESIAN_POINT ( 'NONE',  ( 53.00431643774457768, 93.53749527547704190, -6.986323292181506162 ) ) ;
#15304=AXIS2_PLACEMENT_3D ( 'NONE', #18725, #20495, #13650 ) ;
#15309=CARTESIAN_POINT ( 'NONE',  ( 44.19315180539718568, 85.77372119115894122, -12.70412401877768005 ) ) ;
#15319=CARTESIAN_POINT ( 'NONE',  ( 20.69791174355615837, 145.8831102580302570, -4.951040100860263138 ) ) ;
#15326=CARTESIAN_POINT ( 'NONE',  ( 64.22416581780682066, 138.6102112617928128, -3.133847767204844370 ) ) ;
#15338=CARTESIAN_POINT ( 'NONE',  ( 68.77576173894735234, 108.4446202281264249, 13.13264940013829296 ) ) ;
#15345=CARTESIAN_POINT ( 'NONE',  ( 42.35272797528494237, 144.9004681788466087, 29.24343323619035573 ) ) ;
#15350=CARTESIAN_POINT ( 'NONE',  ( 72.04953363923264931, 101.6246461802091972, -1.784078408812360017 ) ) ;
#15360=CARTESIAN_POINT ( 'NONE',  ( 32.14050509837299785, 87.44534670509604268, 7.696117750009315195 ) ) ;
#15362=CARTESIAN_POINT ( 'NONE',  ( 65.02675087932300357, 102.2843278501921418, -7.581721168364237151 ) ) ;
#15369=CARTESIAN_POINT ( 'NONE',  ( 23.17700876947760591, 147.8092992330439586, -3.851376987104358829 ) ) ;
#15379=CARTESIAN_POINT ( 'NONE',  ( 60.80507725967250821, 98.03074643439879310, -7.343579217248467295 ) ) ;
#15387=CARTESIAN_POINT ( 'NONE',  ( 71.19781441516849441, 139.1947734567256703, -15.08494495145127878 ) ) ;
#15403=CARTESIAN_POINT ( 'NONE',  ( 14.73513546934961482, 119.4163655414939740, 1.151864106104608432 ) ) ;
#15408=CARTESIAN_POINT ( 'NONE',  ( 20.75180444880664510, 93.89949152720284076, -5.875022464008872625 ) ) ;
#15410=CARTESIAN_POINT ( 'NONE',  ( 46.56541826512206228, 91.93282113015048651, 0.2755065429245392439 ) ) ;
#15421=CARTESIAN_POINT ( 'NONE',  ( 51.37827275082728562, 86.79484443300951568, -12.94217320967262275 ) ) ;
#15430=CARTESIAN_POINT ( 'NONE',  ( 15.97061701817242785, 140.8453463817331794, 16.82122940411608170 ) ) ;
#15434=CARTESIAN_POINT ( 'NONE',  ( 15.47577296012077142, 113.4559151263126040, 0.9141320964044082897 ) ) ;
#15435=SURFACE_STYLE_USAGE ( .BOTH. , #1984 ) ;
#15445=CARTESIAN_POINT ( 'NONE',  ( 61.33076419740685736, 141.3451534613812441, 11.70407797152743079 ) ) ;
#15451=CARTESIAN_POINT ( 'NONE',  ( 47.85071283015097521, 95.37984053634411907, 32.91136586774996431 ) ) ;
#15459=CARTESIAN_POINT ( 'NONE',  ( 50.13766412853455279, 153.4730781396112889, -3.927228689826556707 ) ) ;
#15465=CARTESIAN_POINT ( 'NONE',  ( 18.20936163119166196, 143.5026679720446907, 2.934308097026923967 ) ) ;
#15474=CARTESIAN_POINT ( 'NONE',  ( 8.944919112598912037, 123.2842988173194385, -4.803623532975393573 ) ) ;
#15481=CARTESIAN_POINT ( 'NONE',  ( 70.21798013780751546, 127.3226622636268672, -1.629293503064584536 ) ) ;
#15487=DIRECTION ( 'NONE',  ( -0.000000000000000000, -0.000000000000000000, -1.000000000000000000 ) ) ;
#15490=CARTESIAN_POINT ( 'NONE',  ( 32.43765954726634959, 145.6647664193251615, 11.44158087452429129 ) ) ;
#15495=CARTESIAN_POINT ( 'NONE',  ( 15.58850788081759475, 140.2644050767460442, -10.20415289822252980 ) ) ;
#15507=CARTESIAN_POINT ( 'NONE',  ( 64.22416581780682066, 138.6102112617928128, -3.133847767204844370 ) ) ;
#15511=CARTESIAN_POINT ( 'NONE',  ( 16.16624775068580533, 140.9673012293996237, 10.82561872270659009 ) ) ;
#15512=CARTESIAN_POINT ( 'NONE',  ( 53.64127281404707048, 146.0262708631457542, 11.34682183016344403 ) ) ;
#15520=CARTESIAN_POINT ( 'NONE',  ( 33.37504612857446773, 87.14074678364892179, -12.34672919366563981 ) ) ;
#15529=CARTESIAN_POINT ( 'NONE',  ( 18.65831473100296023, 143.8050973582651579, -5.046215916575388150 ) ) ;
#15533=FACE_OUTER_BOUND ( 'NONE', #13371, .T. ) ;
#15534=CARTESIAN_POINT ( 'NONE',  ( 38.01409278319488294, 147.7425775668531003, 9.723292677533123651 ) ) ;
#15542=CIRCLE ( 'NONE', #21547, 10.00000000000000888 ) ;
#15545=CARTESIAN_POINT ( 'NONE',  ( 64.38652456388278722, 138.1782414180340197, -15.12506982898978158 ) ) ;
#15548=CARTESIAN_POINT ( 'NONE',  ( 44.62520010521203062, 144.8567624833121954, 29.46707291594048783 ) ) ;
#15549=CARTESIAN_POINT ( 'NONE',  ( 186.6412678396190472, 201.9535489151380148, 23.27362312593913174 ) ) ;
#15552=CARTESIAN_POINT ( 'NONE',  ( 47.50469609827003836, 95.31385800265883290, 36.42795439419950299 ) ) ;
#15558=CARTESIAN_POINT ( 'NONE',  ( 76.40658810299491677, 127.4365358892444959, 12.33923360994393903 ) ) ;
#15564=CARTESIAN_POINT ( 'NONE',  ( 69.27296957579615366, 97.94681810169329594, -0.6368323762655749842 ) ) ;
#15566=CARTESIAN_POINT ( 'NONE',  ( 22.10153057061799231, 100.9866247252079745, 1.346821830042071566 ) ) ;
#15573=CARTESIAN_POINT ( 'NONE',  ( 50.92548328124963319, 86.60151408976496157, 0.07716523989554470442 ) ) ;
#15577=CARTESIAN_POINT ( 'NONE',  ( 30.08091612619420729, 88.20954595054467973, -6.232194961517499188 ) ) ;
#15589=CARTESIAN_POINT ( 'NONE',  ( 25.43708531585104993, 141.8584285267105827, 4.160929998272084873 ) ) ;
#15604=CARTESIAN_POINT ( 'NONE',  ( 14.54084317601859588, 100.7536435603138756, 21.43002817983359876 ) ) ;
#15607=ORIENTED_EDGE ( 'NONE', *, *, #6812, .T. ) ;
#15609=CARTESIAN_POINT ( 'NONE',  ( 76.20123706073158587, 111.5182621349952257, -8.137091297256032973 ) ) ;
#15610=CARTESIAN_POINT ( 'NONE',  ( 28.62772086389876947, 95.65184626908498444, 8.013395860235284829 ) ) ;
#15619=CARTESIAN_POINT ( 'NONE',  ( 36.18411527879869993, 86.44273942418264767, -5.442340506565031433 ) ) ;
#15629=CARTESIAN_POINT ( 'NONE',  ( 30.90322180743143576, 151.9278386122780375, 10.43433729856376502 ) ) ;
#15634=CYLINDRICAL_SURFACE ( 'NONE', #13795, 2.999999999999997780 ) ;
#15636=CARTESIAN_POINT ( 'NONE',  ( 16.41399813444308364, 129.5198218381110564, 15.55674365125313763 ) ) ;
#15640=FACE_OUTER_BOUND ( 'NONE', #20561, .T. ) ;
#15647=CARTESIAN_POINT ( 'NONE',  ( 65.77248029998415291, 103.2585056976580091, 13.37079068582577435 ) ) ;
#15660=CARTESIAN_POINT ( 'NONE',  ( 58.01262221917386341, 89.04620360302797621, 5.834872140203966495 ) ) ;
#15666=CARTESIAN_POINT ( 'NONE',  ( 76.81974253126139729, 125.2811442093199616, -1.589308178208348910 ) ) ;
#15668=CARTESIAN_POINT ( 'NONE',  ( 55.20039838223064521, 94.47806301326188816, -0.08174959847185196693 ) ) ;
#15676=CARTESIAN_POINT ( 'NONE',  ( 76.79083979644461522, 114.3551126354810492, -1.232281421064668869 ) ) ;
#15688=CARTESIAN_POINT ( 'NONE',  ( 43.01140435219951996, 70.71049967264875136, 34.21067981925357060 ) ) ;
#15695=CARTESIAN_POINT ( 'NONE',  ( 21.13084688720937976, 146.0403058103794649, -16.94226050084479596 ) ) ;
#15697=DIRECTION ( 'NONE',  ( -1.000000000000000000, 0.000000000000000000, 0.000000000000000000 ) ) ;
#15717=CARTESIAN_POINT ( 'NONE',  ( 47.04142330690687857, 147.8988775214238842, 10.08059930640748902 ) ) ;
#15723=CARTESIAN_POINT ( 'NONE',  ( 44.41273964558330789, 85.70220254879866673, -6.708519844216274564 ) ) ;
#15725=CARTESIAN_POINT ( 'NONE',  ( 23.35610682547305927, 99.68565781958278649, 15.27541961222430444 ) ) ;
#15728=AXIS2_PLACEMENT_3D ( 'NONE', #20777, #2467, #15697 ) ;
#15734=CARTESIAN_POINT ( 'NONE',  ( 76.55129369653414528, 113.4641082036936837, -0.2041528983002713349 ) ) ;
#15743=CARTESIAN_POINT ( 'NONE',  ( 9.203281625063985061, 114.5318647093721864, 15.91056058043385413 ) ) ;
#15748=DIRECTION ( 'NONE',  ( 0.000000000000000000, 0.000000000000000000, 1.000000000000000000 ) ) ;
#15750=CARTESIAN_POINT ( 'NONE',  ( 52.07920593110389262, 93.11959619657488929, 13.05671643426689776 ) ) ;
#15759=CARTESIAN_POINT ( 'NONE',  ( 24.14732448757077776, 99.05405632904258084, -4.767757741039170938 ) ) ;
#15766=CARTESIAN_POINT ( 'NONE',  ( 47.34189385015955054, 95.28487160918048460, 31.70594869545381655 ) ) ;
#15772=CARTESIAN_POINT ( 'NONE',  ( 40.23585178891228509, 85.70481357498144348, 6.429941473113898631 ) ) ;
#15779=CARTESIAN_POINT ( 'NONE',  ( 59.83664469576316236, 97.27638873328486113, 6.703993115985443119 ) ) ;
#15785=CARTESIAN_POINT ( 'NONE',  ( 55.11952973528949684, 87.88698225678692211, -7.065691903092018222 ) ) ;
#15794=CARTESIAN_POINT ( 'NONE',  ( 54.54805624998882507, 152.1374805055981199, -2.779977617235711129 ) ) ;
#15800=CARTESIAN_POINT ( 'NONE',  ( 17.98086284713512129, 132.6641746743869135, 10.68742175872072409 ) ) ;
#15817=CARTESIAN_POINT ( 'NONE',  ( 46.79023103138236905, 91.88018867020078062, 6.271112617211819007 ) ) ;
#15822=CARTESIAN_POINT ( 'NONE',  ( 55.11952973528949684, 87.88698225678692211, -7.065691903092018222 ) ) ;
#15824=CARTESIAN_POINT ( 'NONE',  ( 33.01799438418878907, 146.2770090272405810, 10.51364782838779099 ) ) ;
#15831=EDGE_CURVE ( 'NONE', #5848, #18715, #5694, .T. ) ;
#15835=CARTESIAN_POINT ( 'NONE',  ( 35.49642027120339094, 86.59030162945495590, 1.581590266896775843 ) ) ;
#15837=CARTESIAN_POINT ( 'NONE',  ( 15.97061701817242785, 140.8453463817331794, 16.82122940411608170 ) ) ;
#15843=CARTESIAN_POINT ( 'NONE',  ( 61.83586340360074018, 91.21788411573329824, -1.307985002297802568 ) ) ;
#15845=DIRECTION ( 'NONE',  ( 0.9387810623359077455, 0.3426822732243068881, 0.03548206049944094276 ) ) ;
#15848=DIRECTION ( 'NONE',  ( 1.000000000000000000, 0.000000000000000000, 0.000000000000000000 ) ) ;
#15849=CARTESIAN_POINT ( 'NONE',  ( 49.77943037783704483, 92.44786530929899016, 6.152137702922222395 ) ) ;
#15861=CARTESIAN_POINT ( 'NONE',  ( 22.77429378292968920, 139.4308542021594519, -2.981927144630473148 ) ) ;
#15868=LINE ( 'NONE', #20956, #14690 ) ;
#15873=CARTESIAN_POINT ( 'NONE',  ( 11.68597903420391226, 105.9017562933008918, 7.620467510411443435 ) ) ;
#15879=CARTESIAN_POINT ( 'NONE',  ( 71.16904767199986281, 118.3707548728134213, -1.272037577920760665 ) ) ;
#15887=CARTESIAN_POINT ( 'NONE',  ( 77.22939692449374149, 120.9137088693742044, 5.553548964694690504 ) ) ;
#15897=CARTESIAN_POINT ( 'NONE',  ( 8.779377865064803999, 119.6051361893432130, -4.922546661887801100 ) ) ;
#15904=CARTESIAN_POINT ( 'NONE',  ( 60.78979090282389564, 90.74622564588611340, -6.275468401765792237 ) ) ;
#15910=( GEOMETRIC_REPRESENTATION_CONTEXT ( 3 ) GLOBAL_UNCERTAINTY_ASSIGNED_CONTEXT ( ( #18781 ) ) GLOBAL_UNIT_ASSIGNED_CONTEXT ( ( #10190, #13586, #13696 ) ) REPRESENTATION_CONTEXT ( 'NONE', 'WORKASPACE' ) );
#15924=CARTESIAN_POINT ( 'NONE',  ( 14.90453237821946253, 123.0362832886413855, 8.294721248935834623 ) ) ;
#15931=CARTESIAN_POINT ( 'NONE',  ( 57.78275410301085913, 89.02518083909171764, -0.1607367497116551913 ) ) ;
#15932=CARTESIAN_POINT ( 'NONE',  ( 16.56453993303484395, 129.6948329502664308, 9.561135973024818213 ) ) ;
#15933=DIRECTION ( 'NONE',  ( 0.7066505893342460709, 0.7066505893340065958, 0.03591502732094191408 ) ) ;
#15943=CARTESIAN_POINT ( 'NONE',  ( 10.18435502709129103, 110.4832086711448227, 2.772112504659519416 ) ) ;
#15945=CARTESIAN_POINT ( 'NONE',  ( 30.90322180743143576, 151.9278386122780375, 10.43433729856376502 ) ) ;
#15956=CARTESIAN_POINT ( 'NONE',  ( 54.90439719837324617, 94.24896709312837118, 12.93774216356182372 ) ) ;
#15966=CARTESIAN_POINT ( 'NONE',  ( 64.45983652262509622, 101.7220219035630748, -6.553643814208265361 ) ) ;
#15975=CARTESIAN_POINT ( 'NONE',  ( 18.86674891209846905, 143.9013856721611546, -11.04182128657428485 ) ) ;
#15981=CARTESIAN_POINT ( 'NONE',  ( 30.25101221841200427, 88.05347211559326581, -0.2365872832861977970 ) ) ;
#15987=CARTESIAN_POINT ( 'NONE',  ( 56.80456144658707274, 95.31062238922963559, 13.84685026556700116 ) ) ;
#15995=CARTESIAN_POINT ( 'NONE',  ( 77.07719282571002850, 116.5297446719512209, 12.69640610750513865 ) ) ;
#16004=CARTESIAN_POINT ( 'NONE',  ( 30.08091612619420729, 88.20954595054467973, -6.232194961517499188 ) ) ;
#16027=CARTESIAN_POINT ( 'NONE',  ( 43.42882498487155374, 148.1844126167958393, 2.937742163556189112 ) ) ;
#16033=CARTESIAN_POINT ( 'NONE',  ( 13.78455932396994577, 137.7305411390292420, 2.696406107442721467 ) ) ;
#16034=CARTESIAN_POINT ( 'NONE',  ( 40.94005093944240059, 91.86375568685591020, -12.50564155961141566 ) ) ;
#16035=CARTESIAN_POINT ( 'NONE',  ( 23.17700876947760591, 147.8092992330439586, -3.851376987104358829 ) ) ;
#16048=CARTESIAN_POINT ( 'NONE',  ( 60.78979090282389564, 90.74622564588611340, -6.275468401765792237 ) ) ;
#16057=CARTESIAN_POINT ( 'NONE',  ( 76.86499250339331013, 125.5074929390188316, 4.406300711698651895 ) ) ;
#16061=DIRECTION ( 'NONE',  ( 1.000000000000000000, 0.000000000000000000, 0.000000000000000000 ) ) ;
#16064=CARTESIAN_POINT ( 'NONE',  ( 48.57925227495098852, 92.17995633088730756, 20.19957357060707182 ) ) ;
#16076=CARTESIAN_POINT ( 'NONE',  ( 50.40261314387542768, 147.0381507142914188, -1.791644202716362821 ) ) ;
#16086=CARTESIAN_POINT ( 'NONE',  ( 10.42839491720816625, 130.4056617841633283, -4.565575592310756825 ) ) ;
#16093=CARTESIAN_POINT ( 'NONE',  ( 63.99609067623438108, 147.0574274800572425, 3.572798616028722396 ) ) ;
#16094=AXIS2_PLACEMENT_3D ( 'NONE', #8483, #1854, #21814 ) ;
#16095=ORIENTED_EDGE ( 'NONE', *, *, #12715, .T. ) ;
#16100=CARTESIAN_POINT ( 'NONE',  ( 63.85057544308668298, 100.9084186779620609, 13.48995955233852229 ) ) ;
#16113=CARTESIAN_POINT ( 'NONE',  ( 55.94180145820917716, 151.6039095241057453, 11.26783467880839140 ) ) ;
#16122=CARTESIAN_POINT ( 'NONE',  ( 8.944919112598912037, 123.2842988173194385, -4.803623532975393573 ) ) ;
#16144=CARTESIAN_POINT ( 'NONE',  ( 52.31916092102454741, 146.6125112339981627, 3.294994845742023948 ) ) ;
#16150=CARTESIAN_POINT ( 'NONE',  ( 57.94507594753278568, 150.7106492751291569, -2.660852849641732298 ) ) ;
#16151=CARTESIAN_POINT ( 'NONE',  ( 34.95631105476920197, 146.8486248254830855, -9.410786671241964996 ) ) ;
#16152=CARTESIAN_POINT ( 'NONE',  ( 43.80529445460960858, 154.1304981347762748, -3.137004163733609907 ) ) ;
#16160=CARTESIAN_POINT ( 'NONE',  ( 9.997522862669264043, 111.1595821513141402, 9.795857695845493041 ) ) ;
#16163=CARTESIAN_POINT ( 'NONE',  ( 62.34613790317991544, 148.1570561279473850, 11.50573666851796339 ) ) ;
#16168=CARTESIAN_POINT ( 'NONE',  ( 11.58389279593228238, 133.6817500236834917, 1.549157854527217104 ) ) ;
#16175=CARTESIAN_POINT ( 'NONE',  ( 57.39747520560054284, 144.1616143014069280, -9.486357586414486676 ) ) ;
#16185=CARTESIAN_POINT ( 'NONE',  ( 17.40773937504753377, 131.5336607133424991, -10.36307277412196903 ) ) ;
#16193=CARTESIAN_POINT ( 'NONE',  ( 55.11952973528949684, 87.88698225678692211, -7.065691903092018222 ) ) ;
#16200=CARTESIAN_POINT ( 'NONE',  ( 43.13803657676253067, 85.59359249887060628, 13.33475322466254198 ) ) ;
#16217=CARTESIAN_POINT ( 'NONE',  ( 38.54497605562327323, 85.96704844161884296, 14.48200433579215662 ) ) ;
#16225=CARTESIAN_POINT ( 'NONE',  ( 51.78234217841457365, 152.9971814535558963, 4.124977536042813142 ) ) ;
#16252=CARTESIAN_POINT ( 'NONE',  ( 68.93731127356984700, 108.6095829621005180, 19.12825547442421126 ) ) ;
#16258=CARTESIAN_POINT ( 'NONE',  ( 76.79083979644461522, 114.3551126354810492, -1.232281421064668869 ) ) ;
#16259=CARTESIAN_POINT ( 'NONE',  ( 58.12682455153977656, 96.19528378222683784, -13.22021563155647428 ) ) ;
#16270=CARTESIAN_POINT ( 'NONE',  ( 28.88048086162541850, 151.0887240815949895, -10.63664014359656385 ) ) ;
#16279=CARTESIAN_POINT ( 'NONE',  ( 71.48324150724619130, 139.0594858779678873, 3.930207297951037848 ) ) ;
#16285=CARTESIAN_POINT ( 'NONE',  ( 49.02192908010439254, 147.4586317741252799, -9.843465619175002956 ) ) ;
#16294=CARTESIAN_POINT ( 'NONE',  ( 21.63557314705429846, 101.6375443364048152, 2.375099401820868206 ) ) ;
#16302=CARTESIAN_POINT ( 'NONE',  ( 43.80529445460960858, 154.1304981347762748, -3.137004163733609907 ) ) ;
#16309=CARTESIAN_POINT ( 'NONE',  ( 19.22998607435487273, 95.16999353120945671, 21.19198650444592857 ) ) ;
#16313=CARTESIAN_POINT ( 'NONE',  ( 20.11427441861009058, 94.56644311770523359, -4.846896973145477183 ) ) ;
#16316=CARTESIAN_POINT ( 'NONE',  ( 23.35610682547305927, 99.68565781958278649, 15.27541961222430444 ) ) ;
#16321=CARTESIAN_POINT ( 'NONE',  ( 70.74141321743030630, 114.7826485538520416, 5.870819564965037429 ) ) ;
#16323=CARTESIAN_POINT ( 'NONE',  ( 62.34613790317991544, 148.1570561279473850, 11.50573666851796339 ) ) ;
#16324=CARTESIAN_POINT ( 'NONE',  ( 39.04181488774997888, 95.22401868161449556, 37.25520735466819389 ) ) ;
#16334=CARTESIAN_POINT ( 'NONE',  ( 61.01612483116806374, 90.79174121657607088, -0.2798613066081144796 ) ) ;
#16348=ADVANCED_FACE ( 'NONE', ( #10741 ), #14595, .T. ) ;
#16358=CARTESIAN_POINT ( 'NONE',  ( 22.30625593121589390, 139.1551866335812235, 23.00981086756132044 ) ) ;
#16364=CARTESIAN_POINT ( 'NONE',  ( 40.90832812944997698, 154.0758954209757121, 3.767805038447253452 ) ) ;
#16366=CARTESIAN_POINT ( 'NONE',  ( 17.81206540393426252, 132.5069038242342003, 16.68302557436956945 ) ) ;
#16382=CARTESIAN_POINT ( 'NONE',  ( 16.10574266336056226, 141.2029798434031989, 15.83487214029357659 ) ) ;
#16388=CARTESIAN_POINT ( 'NONE',  ( 70.00144543033923128, 111.4600545017090241, 19.00928056007509070 ) ) ;
#16400=CARTESIAN_POINT ( 'NONE',  ( 23.25700774553339301, 99.89415360575743819, 9.279811863844059872 ) ) ;
#16408=CARTESIAN_POINT ( 'NONE',  ( 30.18028515090227160, 151.2280014487717779, 17.43780275515692679 ) ) ;
#16412=CARTESIAN_POINT ( 'NONE',  ( 72.98789752971651978, 103.3738663174133023, 6.148623012889737005 ) ) ;
#16418=CARTESIAN_POINT ( 'NONE',  ( 70.82039710638956365, 99.80338443054456832, 19.28708432993385102 ) ) ;
#16421=CARTESIAN_POINT ( 'NONE',  ( 29.91082003397629663, 88.36561978549612206, -12.22780263974880022 ) ) ;
#16424=CARTESIAN_POINT ( 'NONE',  ( 42.37836782381873491, 91.71465960395167372, 14.44224817795539373 ) ) ;
#16429=CARTESIAN_POINT ( 'NONE',  ( 24.25535704844963547, 98.85002770340597067, 1.227849354118501601 ) ) ;
#16436=PRODUCT_DEFINITION_SHAPE ( 'NONE', 'NONE',  #18895 ) ;
#16441=CARTESIAN_POINT ( 'NONE',  ( 14.15704070161504369, 138.3271338521546454, 9.720138693322796897 ) ) ;
#16465=CARTESIAN_POINT ( 'NONE',  ( 24.99951789580824268, 141.7104366081036346, 16.15213770299339657 ) ) ;
#16471=CARTESIAN_POINT ( 'NONE',  ( 18.14018356548558941, 143.3940520581896862, 16.92415443696469879 ) ) ;
#16472=CARTESIAN_POINT ( 'NONE',  ( 15.18239976710701100, 124.4615124019231018, 16.34704286353642999 ) ) ;
#16488=CARTESIAN_POINT ( 'NONE',  ( 55.77169822954404310, 151.7599422098969910, 17.26344356872107255 ) ) ;
#16493=CARTESIAN_POINT ( 'NONE',  ( 31.96084264191244273, 87.59053552682176758, 1.700516636338098797 ) ) ;
#16494=CARTESIAN_POINT ( 'NONE',  ( 43.06284635655732274, 148.1064719378950088, -10.08176808973812655 ) ) ;
#16506=CARTESIAN_POINT ( 'NONE',  ( 14.94553207812311690, 121.6546367895698779, 10.23235069918434981 ) ) ;
#16517=CARTESIAN_POINT ( 'NONE',  ( 73.32203938827501588, 103.9946350594383517, -0.8753108214479579097 ) ) ;
#16524=CARTESIAN_POINT ( 'NONE',  ( 73.69864372527810303, 135.2613471474284097, 11.07306444099484466 ) ) ;
#16527=CARTESIAN_POINT ( 'NONE',  ( 71.68162264554656815, 101.3460857334412708, -13.77530061520655025 ) ) ;
#16538=CARTESIAN_POINT ( 'NONE',  ( 17.48807464456866256, 131.8965856249792523, 2.656420782620954935 ) ) ;
#16540=CARTESIAN_POINT ( 'NONE',  ( 30.18028515090226449, 151.2280014487717779, 17.43780275515692679 ) ) ;
#16550=CARTESIAN_POINT ( 'NONE',  ( 67.39040179371399120, 143.9404232637865562, 4.720051584306741432 ) ) ;
#16557=CARTESIAN_POINT ( 'NONE',  ( 74.62708615766334219, 133.0342049366344384, -8.851289726714327344 ) ) ;
#16573=CARTESIAN_POINT ( 'NONE',  ( 65.96530660583994177, 103.3855952397044007, 19.36639486037446289 ) ) ;
#16579=CARTESIAN_POINT ( 'NONE',  ( 14.48810111090402941, 100.9784058478479523, 15.43442115621699529 ) ) ;
#16580=CARTESIAN_POINT ( 'NONE',  ( 69.09677972725788209, 109.4046064338026127, -6.910527774811301427 ) ) ;
#16601=CARTESIAN_POINT ( 'NONE',  ( 74.43934690056714487, 106.1333445020626129, 19.04903893889577660 ) ) ;
#16608=CARTESIAN_POINT ( 'NONE',  ( 62.62098228421420032, 91.94359626243755201, 7.653270806628301948 ) ) ;
#16610=CARTESIAN_POINT ( 'NONE',  ( 15.00983914341701997, 123.2415857317943448, 2.299110145932334426 ) ) ;
#16622=CARTESIAN_POINT ( 'NONE',  ( 45.76500403897348690, 91.92250713676531859, 1.303787141088997181 ) ) ;
#16633=CARTESIAN_POINT ( 'NONE',  ( 73.40451243997107156, 135.6611253642151098, -1.946480675884423084 ) ) ;
#16641=CARTESIAN_POINT ( 'NONE',  ( 9.691656460246418803, 128.1079710775123601, 15.35877872671195910 ) ) ;
#16644=CARTESIAN_POINT ( 'NONE',  ( 9.647618190908266556, 112.6042302384299916, -11.15662622088235167 ) ) ;
#16652=CARTESIAN_POINT ( 'NONE',  ( 55.20039838223064521, 94.47806301326188816, -0.08174959847185196693 ) ) ;
#16665=CARTESIAN_POINT ( 'NONE',  ( 17.60877916486148465, 96.95950790538488206, 1.267834678905774393 ) ) ;
#16671=CARTESIAN_POINT ( 'NONE',  ( 8.779377865064803999, 119.6051361893432130, -4.922546661887801100 ) ) ;
#16673=CARTESIAN_POINT ( 'NONE',  ( 44.18632541912793243, 91.73153706005567187, -6.629209314582290347 ) ) ;
#16679=CARTESIAN_POINT ( 'NONE',  ( 63.55746018358933469, 147.2895578332197033, -9.446739241148069510 ) ) ;
#16680=CARTESIAN_POINT ( 'NONE',  ( 23.10700517764655260, 139.6571016847272801, -10.96257334342637435 ) ) ;
#16689=CARTESIAN_POINT ( 'NONE',  ( 15.78326802858598299, 112.2624592280589439, 21.86641499745291028 ) ) ;
#16696=CARTESIAN_POINT ( 'NONE',  ( 9.822352152143091431, 128.2981216602131553, 9.363167623699879982 ) ) ;
#16698=CARTESIAN_POINT ( 'NONE',  ( 33.89447768034496278, 93.30632465966320410, 1.780072726204736000 ) ) ;
#16714=CARTESIAN_POINT ( 'NONE',  ( 73.16288888369128074, 103.5245705370889766, 12.14422718744263285 ) ) ;
#16719=CARTESIAN_POINT ( 'NONE',  ( 34.72595348466361287, 146.8618156516888291, -3.415175568290148345 ) ) ;
#16728=FACE_OUTER_BOUND ( 'NONE', #20966, .T. ) ;
#16731=CARTESIAN_POINT ( 'NONE',  ( 65.91867393726404600, 103.5983250578868109, 0.3515012976045437387 ) ) ;
#16742=CARTESIAN_POINT ( 'NONE',  ( 53.71239221804358976, 87.38980250447106357, 6.982120393166105998 ) ) ;
#16750=CARTESIAN_POINT ( 'NONE',  ( 21.96620680132455306, 138.7984961796735490, 1.985398331534963923 ) ) ;
#16751=DIRECTION ( 'NONE',  ( 1.000000000000000000, 0.000000000000000000, 0.000000000000000000 ) ) ;
#16756=ORIENTED_EDGE ( 'NONE', *, *, #8065, .F. ) ;
#16762=CARTESIAN_POINT ( 'NONE',  ( 15.38454125381035098, 114.2504036285165654, 1.942219256913226388 ) ) ;
#16767=CARTESIAN_POINT ( 'NONE',  ( 43.01140435219951996, 94.90707761860558378, 29.21067981925357060 ) ) ;
#16777=CARTESIAN_POINT ( 'NONE',  ( 74.61827669547474784, 133.2649018527303895, -2.855682626312802785 ) ) ;
#16783=CARTESIAN_POINT ( 'NONE',  ( 68.88151390383544026, 142.3271613368909811, -9.208263745312144977 ) ) ;
#16786=CARTESIAN_POINT ( 'NONE',  ( 71.13433436327568415, 121.9840874124550965, -8.414894741535439593 ) ) ;
#16791=CARTESIAN_POINT ( 'NONE',  ( 18.35401747797491723, 143.4883766228698221, 10.92869415326320670 ) ) ;
#16799=CARTESIAN_POINT ( 'NONE',  ( 14.81332417359726783, 119.6334487847019403, -4.843746996953559147 ) ) ;
#16806=CARTESIAN_POINT ( 'NONE',  ( 9.976645104453018220, 110.9295780357170571, 15.79146183154218619 ) ) ;
#16808=CARTESIAN_POINT ( 'NONE',  ( 15.42009695863806229, 114.4785911120537634, -4.053384917639696994 ) ) ;
#16824=CARTESIAN_POINT ( 'NONE',  ( 11.87357267856223864, 134.3244722033052767, 8.572888645784400907 ) ) ;
#16829=CARTESIAN_POINT ( 'NONE',  ( 76.55129369653414528, 113.4641082036936837, -0.2041528983002713349 ) ) ;
#16831=CARTESIAN_POINT ( 'NONE',  ( 26.65597624659334031, 142.8797025615743337, -3.772066457372480475 ) ) ;
#16841=CARTESIAN_POINT ( 'NONE',  ( 76.02541712503827398, 128.6535784478189726, -7.704039830276845358 ) ) ;
#16848=CARTESIAN_POINT ( 'NONE',  ( 69.27296957579615366, 97.94681810169329594, -0.6368323762655749842 ) ) ;
#16856=CARTESIAN_POINT ( 'NONE',  ( 27.23529593042425390, 96.43589704216468306, 0.08059930645588880838 ) ) ;
#16869=CARTESIAN_POINT ( 'NONE',  ( 26.83015598135647295, 142.9878415585355071, 17.22988066553158149 ) ) ;
#16881=CARTESIAN_POINT ( 'NONE',  ( 23.00888394656308122, 147.7027690514567837, -4.855972970016076751 ) ) ;
#16889=CARTESIAN_POINT ( 'NONE',  ( 75.80354157443048280, 110.0810758630161672, 5.910575721798123183 ) ) ;
#16891=CARTESIAN_POINT ( 'NONE',  ( 34.17400395940548918, 146.6865494356538875, -10.43883331896520694 ) ) ;
#16897=CARTESIAN_POINT ( 'NONE',  ( 16.50170782505827560, 141.4403336307199197, 3.843654360456687513 ) ) ;
#16908=CARTESIAN_POINT ( 'NONE',  ( 60.38095089740433252, 142.1228462996803046, -2.343495028824083004 ) ) ;
#16915=CARTESIAN_POINT ( 'NONE',  ( 42.21854335081802390, 85.68333463812091111, 14.36287948008016890 ) ) ;
#16916=CARTESIAN_POINT ( 'NONE',  ( 57.63517438308760177, 95.88943085326536675, -6.196329169593343345 ) ) ;
#16917=MECHANICAL_DESIGN_GEOMETRIC_PRESENTATION_REPRESENTATION('',(#14803),#14095);
#16930=CARTESIAN_POINT ( 'NONE',  ( 66.11232864078046134, 136.2219195394164899, -3.014685448219384334 ) ) ;
#16934=CARTESIAN_POINT ( 'NONE',  ( 73.74613032677598312, 134.8023270448005064, -0.9181577650121128809 ) ) ;
#16935=CARTESIAN_POINT ( 'NONE',  ( 70.85748824340309682, 124.3570181999574515, -1.510321027129504889 ) ) ;
#16944=CARTESIAN_POINT ( 'NONE',  ( 63.68221904981356829, 147.0951523173380338, -15.44234037292825690 ) ) ;
#16957=CARTESIAN_POINT ( 'NONE',  ( 68.29446192123552350, 96.82662215664792882, 13.41040346623746515 ) ) ;
#16963=CARTESIAN_POINT ( 'NONE',  ( 16.02160000510927418, 128.3529272436884128, 1.509170735004851549 ) ) ;
#16964=CARTESIAN_POINT ( 'NONE',  ( 43.01140435219951996, 119.9070776186055838, -19.99999999999997868 ) ) ;
#16975=CARTESIAN_POINT ( 'NONE',  ( 69.30627838890079317, 109.9422389716749535, -13.93421298911417416 ) ) ;
#16983=CARTESIAN_POINT ( 'NONE',  ( 39.24503612293847254, 144.6228301878137188, 37.51526355657936307 ) ) ;
#16989=CARTESIAN_POINT ( 'NONE',  ( 71.08298874133512868, 139.6419663798271529, -3.093729572736475752 ) ) ;
#16994=CARTESIAN_POINT ( 'NONE',  ( 66.24914683137549787, 94.76885710642066840, 6.506024766557033878 ) ) ;
#17003=EDGE_CURVE ( 'NONE', #4221, #1853, #15542, .T. ) ;
#17004=CARTESIAN_POINT ( 'NONE',  ( 26.90790578767411390, 150.1165885900122987, 3.291480155758420345 ) ) ;
#17014=CARTESIAN_POINT ( 'NONE',  ( 27.10205971394288582, 96.62443569844734270, -5.915007788698968483 ) ) ;
#17022=CARTESIAN_POINT ( 'NONE',  ( 45.76500403897348690, 91.92250713676531859, 1.303787141088997181 ) ) ;
#17027=AXIS2_PLACEMENT_3D ( 'NONE', #2701, #9331, #1055 ) ;
#17039=CARTESIAN_POINT ( 'NONE',  ( 70.07576047146775977, 128.1116393178318731, -2.657569147260473663 ) ) ;
#17043=CARTESIAN_POINT ( 'NONE',  ( 40.73010619540765020, 85.74955863377461185, -6.589596535617429751 ) ) ;
#17044=CARTESIAN_POINT ( 'NONE',  ( 68.03731475862628031, 132.9047928164914367, -1.867435455408581912 ) ) ;
#17055=CARTESIAN_POINT ( 'NONE',  ( 64.23777839346797691, 146.6638261710672566, -8.418409733082999225 ) ) ;
#17064=CARTESIAN_POINT ( 'NONE',  ( 8.829984022807513711, 121.7968051057545580, 16.14860047415989541 ) ) ;
#17069=CARTESIAN_POINT ( 'NONE',  ( 71.28213884770818254, 119.1643779896719764, -2.300315981272657240 ) ) ;
#17071=DIRECTION ( 'NONE',  ( 0.000000000000000000, 0.000000000000000000, 1.000000000000000000 ) ) ;
#17082=CARTESIAN_POINT ( 'NONE',  ( 14.85320491933239317, 121.4429315054255909, 16.22795414098078126 ) ) ;
#17088=CARTESIAN_POINT ( 'NONE',  ( 43.34266540673962709, 94.90707761860556957, 39.21067981925357060 ) ) ;
#17090=CARTESIAN_POINT ( 'NONE',  ( 42.68462674639443577, 144.9070776186055980, 29.21067981925357770 ) ) ;
#17095=CARTESIAN_POINT ( 'NONE',  ( 26.66797635711824199, 149.9459070286683868, 17.30505193804556185 ) ) ;
#17101=CARTESIAN_POINT ( 'NONE',  ( 13.33420504782278293, 102.8437529505761603, 1.505736668420971869 ) ) ;
#17103=CARTESIAN_POINT ( 'NONE',  ( 27.10205971394288582, 96.62443569844734270, -5.915007788698968483 ) ) ;
#17111=CARTESIAN_POINT ( 'NONE',  ( 36.38086904327614235, 86.32171732562966326, 0.5532606071062302622 ) ) ;
#17118=AXIS2_PLACEMENT_3D ( 'NONE', #19485, #21150, #16061 ) ;
#17122=CARTESIAN_POINT ( 'NONE',  ( 69.45715107853048664, 110.1171555912624740, -7.938611875467805667 ) ) ;
#17130=CARTESIAN_POINT ( 'NONE',  ( 54.06307869441068448, 152.2224424482157303, -15.79932498977872868 ) ) ;
#17148=CARTESIAN_POINT ( 'NONE',  ( 26.43292637418678126, 142.8198486544370098, 2.223537717183381002 ) ) ;
#17152=CARTESIAN_POINT ( 'NONE',  ( 77.22348061889915982, 118.7203125366680752, -8.375138532479306619 ) ) ;
#17153=CARTESIAN_POINT ( 'NONE',  ( 25.21830160582964453, 141.7844325674071229, 10.15653385063274428 ) ) ;
#17164=CARTESIAN_POINT ( 'NONE',  ( 66.98923854426821833, 144.2286169274386509, -8.299483363615854259 ) ) ;
#17169=DIRECTION ( 'NONE',  ( 1.000000000000000000, 0.000000000000000000, 0.000000000000000000 ) ) ;
#17174=CARTESIAN_POINT ( 'NONE',  ( 38.54497605562327323, 85.96704844161884296, 14.48200433579215662 ) ) ;
#17179=CARTESIAN_POINT ( 'NONE',  ( 14.87688376430095616, 117.0300574687981481, 8.056989239287382532 ) ) ;
#17189=CARTESIAN_POINT ( 'NONE',  ( 34.40470276422951912, 146.6778736915268553, -16.43444041970612446 ) ) ;
#17191=CARTESIAN_POINT ( 'NONE',  ( 45.07664058499605630, 144.8220846865936551, 29.65421901078121536 ) ) ;
#17200=CARTESIAN_POINT ( 'NONE',  ( 59.73150498404358899, 90.03452709159309109, 13.76780503130795097 ) ) ;
#17205=CARTESIAN_POINT ( 'NONE',  ( 77.22939692449374149, 120.9137088693742044, 5.553548964694690504 ) ) ;
#17208=CARTESIAN_POINT ( 'NONE',  ( 19.85370653151704090, 103.8158566922722486, 8.489678972899794118 ) ) ;
#17215=CARTESIAN_POINT ( 'NONE',  ( 32.98198692859195802, 152.6383102900375093, -3.493975233523312962 ) ) ;
#17220=CARTESIAN_POINT ( 'NONE',  ( 10.61900875472251649, 108.8314319666055212, -5.279948415675857376 ) ) ;
#17229=ORIENTED_EDGE ( 'NONE', *, *, #15831, .F. ) ;
#17233=CARTESIAN_POINT ( 'NONE',  ( 63.68221904981356829, 147.0951523173380338, -15.44234037292825690 ) ) ;
#17252=CARTESIAN_POINT ( 'NONE',  ( 42.43310160994198554, 85.59785666124599857, 20.35848333119881914 ) ) ;
#17258=CARTESIAN_POINT ( 'NONE',  ( 12.60192345832597027, 135.3850619972812979, 10.60811072801600119 ) ) ;
#17259=CARTESIAN_POINT ( 'NONE',  ( 69.49396330798431620, 129.5978393632817927, 5.275421687385184910 ) ) ;
#17269=CARTESIAN_POINT ( 'NONE',  ( 9.647618190908266556, 112.6042302384299916, -11.15662622088235167 ) ) ;
#17279=CARTESIAN_POINT ( 'NONE',  ( 76.40658810299491677, 127.4365358892444959, 12.33923360994393903 ) ) ;
#17285=CARTESIAN_POINT ( 'NONE',  ( 15.40311202476076780, 126.0397005259128065, 8.413886508562818278 ) ) ;
#17298=CARTESIAN_POINT ( 'NONE',  ( 48.35156950851215640, 92.21792820573091376, 14.20396468032920012 ) ) ;
#17300=CARTESIAN_POINT ( 'NONE',  ( 46.98624069623303967, 144.5897511595969149, 31.15999777443385810 ) ) ;
#17311=CARTESIAN_POINT ( 'NONE',  ( 66.79148812173782801, 144.6461433805978061, 3.691718863876278345 ) ) ;
#17313=CIRCLE ( 'NONE', #9589, 3.000000000000000444 ) ;
#17315=AXIS2_PLACEMENT_3D ( 'NONE', #20506, #15748, #15848 ) ;
#17318=CARTESIAN_POINT ( 'NONE',  ( 50.92548328124963319, 86.60151408976496157, 0.07716523989554470442 ) ) ;
#17321=CARTESIAN_POINT ( 'NONE',  ( 66.49460585200260709, 135.5194395740885511, -1.986604139701473759 ) ) ;
#17330=CARTESIAN_POINT ( 'NONE',  ( 23.67598417054553295, 91.65793073385727041, -5.994147020910363999 ) ) ;
#17340=CARTESIAN_POINT ( 'NONE',  ( 77.22348061889915982, 118.7203125366680752, -8.375138532479306619 ) ) ;
#17345=CARTESIAN_POINT ( 'NONE',  ( 39.14927582833848874, 92.05416703502255871, 8.565614722876343734 ) ) ;
#17355=EDGE_CURVE ( 'NONE', #10804, #11596, #21184, .T. ) ;
#17363=CARTESIAN_POINT ( 'NONE',  ( 66.29928749942908439, 103.8601778506706239, 12.34270352495849110 ) ) ;
#17368=CARTESIAN_POINT ( 'NONE',  ( 32.98198692859195802, 152.6383102900375093, -3.493975233523312962 ) ) ;
#17370=CARTESIAN_POINT ( 'NONE',  ( 30.72731853479779929, 94.52359049060457608, 14.91853181686295038 ) ) ;
#17378=CARTESIAN_POINT ( 'NONE',  ( 39.81857293680397447, 85.90283706545402254, -5.561266875997713299 ) ) ;
#17388=CARTESIAN_POINT ( 'NONE',  ( 19.13088699441526686, 95.37848931739559077, 15.19637875606281341 ) ) ;
#17396=CARTESIAN_POINT ( 'NONE',  ( 27.44638778410068625, 143.5188605762539851, 16.27111261720311930 ) ) ;
#17406=CARTESIAN_POINT ( 'NONE',  ( 57.63517438308760177, 95.88943085326536675, -6.196329169593343345 ) ) ;
#17408=LINE ( 'NONE', #21771, #13276 ) ;
#17412=CARTESIAN_POINT ( 'NONE',  ( 43.67008072911410466, 94.91368705836457309, 29.24343323619035928 ) ) ;
#17419=CARTESIAN_POINT ( 'NONE',  ( 47.97332496630577481, 153.8600623441721211, 10.00146007428102379 ) ) ;
#17425=CARTESIAN_POINT ( 'NONE',  ( 37.00104444766353851, 92.35499785847434850, 7.656504971210453370 ) ) ;
#17433=CARTESIAN_POINT ( 'NONE',  ( 13.33420504782278293, 102.8437529505761603, 1.505736668420971869 ) ) ;
#17443=CARTESIAN_POINT ( 'NONE',  ( 53.88337135589062399, 152.3674195137575964, -9.803719146365084569 ) ) ;
#17451=CARTESIAN_POINT ( 'NONE',  ( 14.94553207812311690, 121.6546367895698779, 10.23235069918434981 ) ) ;
#17471=CARTESIAN_POINT ( 'NONE',  ( 69.40534582624466964, 109.7482951092767678, 5.080680574306066788 ) ) ;
#17478=CARTESIAN_POINT ( 'NONE',  ( 31.29766364123476663, 87.82482650329993135, 8.724447585906515812 ) ) ;
#17480=CARTESIAN_POINT ( 'NONE',  ( 14.88799800344823154, 117.8296896831652560, 9.085076399755989129 ) ) ;
#17488=CARTESIAN_POINT ( 'NONE',  ( 76.67641731516037851, 114.1545672503790740, -7.227887495354823777 ) ) ;
#17491=CARTESIAN_POINT ( 'NONE',  ( 8.829984022807513711, 121.7968051057545580, 16.14860047415989541 ) ) ;
#17496=CARTESIAN_POINT ( 'NONE',  ( 36.57762280775352082, 86.20069522707665044, 6.548861720777491513 ) ) ;
#17501=CARTESIAN_POINT ( 'NONE',  ( 71.27174135432656499, 120.9783100490299574, 11.62814500561148456 ) ) ;
#17513=CARTESIAN_POINT ( 'NONE',  ( 71.07673676950255981, 118.1590465568689581, -7.267641430287227422 ) ) ;
#17515=DIRECTION ( 'NONE',  ( 0.9387810623359077455, 0.3426822732243072211, 0.03548206049944095664 ) ) ;
#17523=VERTEX_POINT ( 'NONE', #20936 ) ;
#17525=CARTESIAN_POINT ( 'NONE',  ( 17.69433683334896656, 96.74512228834443306, 7.263443568815639573 ) ) ;
#17532=CARTESIAN_POINT ( 'NONE',  ( 45.98873144221455789, 91.86516812052268222, 7.299390993452533394 ) ) ;
#17539=CARTESIAN_POINT ( 'NONE',  ( 46.60148787037231699, 85.86292235506145687, 7.220022382731924537 ) ) ;
#17550=CARTESIAN_POINT ( 'NONE',  ( 76.20123706073158587, 111.5182621349952257, -8.137091297256032973 ) ) ;
#17558=CARTESIAN_POINT ( 'NONE',  ( 73.43285993012185031, 135.4320224564883688, -7.942088354107054826 ) ) ;
#17566=EDGE_CURVE ( 'NONE', #3649, #17523, #5695, .T. ) ;
#17578=CARTESIAN_POINT ( 'NONE',  ( 58.08784223975295902, 95.98046199469133910, 5.794885020722011504 ) ) ;
#17584=CARTESIAN_POINT ( 'NONE',  ( 71.53613896966024299, 138.8348963267899592, -2.065403804986401859 ) ) ;
#17585=CARTESIAN_POINT ( 'NONE',  ( 67.71458430423905384, 106.3058120325361671, 6.227933542621733487 ) ) ;
#17596=CARTESIAN_POINT ( 'NONE',  ( 69.90255027150604406, 140.9627200460241454, -1.156626220813373518 ) ) ;
#17598=CARTESIAN_POINT ( 'NONE',  ( 12.61881386508366809, 104.1535352963828984, 15.55354899318430739 ) ) ;
#17601=CARTESIAN_POINT ( 'NONE',  ( 18.01140435219953062, 119.9070776186055838, 50.00000000000002842 ) ) ;
#17604=CARTESIAN_POINT ( 'NONE',  ( 77.28446211531542076, 118.2294073780637262, 4.644197663618684579 ) ) ;
#17610=CARTESIAN_POINT ( 'NONE',  ( 34.25380259335813093, 93.01594701623474748, 13.77127495354717190 ) ) ;
#17614=COLOUR_RGB ( '', 0.40784314, 0.44705882, 0.49803922) ;
#17615=DIRECTION ( 'NONE',  ( 0.000000000000000000, 0.000000000000000000, -1.000000000000000000 ) ) ;
#17622=CARTESIAN_POINT ( 'NONE',  ( 41.47717036631702570, 147.9855288695934803, -2.148757419388624523 ) ) ;
#17630=CARTESIAN_POINT ( 'NONE',  ( 26.28921445626723852, 149.7786157371718616, -3.732453678475698311 ) ) ;
#17635=CARTESIAN_POINT ( 'NONE',  ( 11.58389279593228238, 133.6817500236834917, 1.549157854527217104 ) ) ;
#17636=ADVANCED_FACE ( 'NONE', ( #15533 ), #15634, .T. ) ;
#17643=CARTESIAN_POINT ( 'NONE',  ( 47.24326884731692644, 147.7868190896643341, 4.084992211255583427 ) ) ;
#17650=CARTESIAN_POINT ( 'NONE',  ( 10.16827731527805767, 110.2528774685086574, 8.767718578943870966 ) ) ;
#17651=CARTESIAN_POINT ( 'NONE',  ( 42.68471116819608113, 94.90707761860558378, 29.21067981925357415 ) ) ;
#17661=CARTESIAN_POINT ( 'NONE',  ( 47.47886434171987702, 153.8471147930492862, -3.017879606865911502 ) ) ;
#17686=CARTESIAN_POINT ( 'NONE',  ( 55.13406075593908895, 145.4575617026882526, 3.413969760132236964 ) ) ;
#17692=CARTESIAN_POINT ( 'NONE',  ( 66.89036333300305159, 144.4373801540182569, -2.303882249869787291 ) ) ;
#17693=CARTESIAN_POINT ( 'NONE',  ( 71.06985403747866314, 121.7623127629220932, -14.41049859375789666 ) ) ;
#17694=CARTESIAN_POINT ( 'NONE',  ( 8.944919112598912037, 123.2842988173194385, -4.803623532975393573 ) ) ;
#17702=CARTESIAN_POINT ( 'NONE',  ( 8.987667018801221985, 116.9306527918008527, -4.013769077970609445 ) ) ;
#17704=CARTESIAN_POINT ( 'NONE',  ( 21.90415124324598750, 92.95514585177724598, 15.07745334355238676 ) ) ;
#17706=( NAMED_UNIT ( * ) SI_UNIT ( $, .STERADIAN. ) SOLID_ANGLE_UNIT ( ) );
#17709=CARTESIAN_POINT ( 'NONE',  ( 76.90526227772885193, 114.5556580205831096, 4.763324653225488703 ) ) ;
#17715=CARTESIAN_POINT ( 'NONE',  ( 16.54882264740998110, 129.8072851447780067, 22.56993813403257931 ) ) ;
#17719=CARTESIAN_POINT ( 'NONE',  ( 43.01140435219951996, 119.9070776186055838, -35.00000000000000000 ) ) ;
#17726=CARTESIAN_POINT ( 'NONE',  ( 49.32098446784893753, 92.50438258598539676, -5.839070001793449372 ) ) ;
#17741=CARTESIAN_POINT ( 'NONE',  ( 26.06094713673110164, 149.7432261477326563, 2.263147435255992601 ) ) ;
#17749=CARTESIAN_POINT ( 'NONE',  ( 35.91077447413180579, 147.1981228300969633, 10.63281669705329691 ) ) ;
#17752=CIRCLE ( 'NONE', #19523, 2.999999999999997780 ) ;
#17757=CARTESIAN_POINT ( 'NONE',  ( 49.46632042442519861, 86.28835692931116341, 14.12497754236212977 ) ) ;
#17758=CARTESIAN_POINT ( 'NONE',  ( 38.94332714213889091, 95.24011124016369934, 37.12229684998503387 ) ) ;
#17766=CARTESIAN_POINT ( 'NONE',  ( 43.80529445460960858, 154.1304981347762748, -3.137004163733609907 ) ) ;
#17768=ORIENTED_EDGE ( 'NONE', *, *, #18588, .T. ) ;
#17777=CARTESIAN_POINT ( 'NONE',  ( 18.01140435219953062, 119.9070776186055838, -19.99999999999997868 ) ) ;
#17790=CARTESIAN_POINT ( 'NONE',  ( 67.88957565821384321, 106.4565162521658976, 12.22353771717463466 ) ) ;
#17796=CARTESIAN_POINT ( 'NONE',  ( 71.03835150376274044, 100.2492380157770526, 6.267546321443639989 ) ) ;
#17797=CARTESIAN_POINT ( 'NONE',  ( 20.50804704269433998, 103.0453634090187762, -11.55335571609641399 ) ) ;
#17798=CARTESIAN_POINT ( 'NONE',  ( 9.616596702810701558, 112.3753283828585694, -5.161025107254184618 ) ) ;
#17807=CARTESIAN_POINT ( 'NONE',  ( 56.91482361236938203, 88.71218622616480332, 0.8673887411229855848 ) ) ;
#17811=CARTESIAN_POINT ( 'NONE',  ( 16.30372524420941716, 141.3216567370616019, 9.839263250375132941 ) ) ;
#17816=CARTESIAN_POINT ( 'NONE',  ( 63.99609067623438108, 147.0574274800572425, 3.572798616028722396 ) ) ;
#17826=CARTESIAN_POINT ( 'NONE',  ( 22.30625593121589390, 139.1551866335812235, 23.00981086756132044 ) ) ;
#17837=CARTESIAN_POINT ( 'NONE',  ( 43.85786119575681852, 148.0137586191354444, -9.053472026759274982 ) ) ;
#17839=DIRECTION ( 'NONE',  ( -0.3428981916074304581, 0.9393725726208712601, 0.000000000000000000 ) ) ;
#17846=CARTESIAN_POINT ( 'NONE',  ( 11.74529739132928619, 133.8467647624810581, -4.446451035385589279 ) ) ;
#17852=CARTESIAN_POINT ( 'NONE',  ( 71.22865828484523831, 100.3801644121689094, 12.26314743512348926 ) ) ;
#17866=CARTESIAN_POINT ( 'NONE',  ( 42.21854335081802390, 85.68333463812091111, 14.36287948008016890 ) ) ;
#17867=CARTESIAN_POINT ( 'NONE',  ( 41.39760859918703062, 94.95739275389902900, 29.46707291594048428 ) ) ;
#17874=CARTESIAN_POINT ( 'NONE',  ( 8.927628897234525240, 116.7075971571176751, 1.981832035706394546 ) ) ;
#17898=CARTESIAN_POINT ( 'NONE',  ( 33.70380864093198170, 93.20109254516876263, 20.79496611990781929 ) ) ;
#17904=CARTESIAN_POINT ( 'NONE',  ( 74.85601106972485752, 107.3429126181175661, -0.9942341299615756745 ) ) ;
#17906=CARTESIAN_POINT ( 'NONE',  ( 23.31543935874208273, 139.7533899986231916, -16.95817871342526573 ) ) ;
#17915=CARTESIAN_POINT ( 'NONE',  ( 20.91437931538276374, 145.9617080342048894, -10.94665030085253044 ) ) ;
#17925=CARTESIAN_POINT ( 'NONE',  ( 8.701189160817120793, 119.3880529461122109, 1.073064441167490557 ) ) ;
#17930=CARTESIAN_POINT ( 'NONE',  ( 53.47116958538193643, 146.1823035489369715, 17.34243072007611985 ) ) ;
#17939=CLOSED_SHELL ( 'NONE', ( #11191, #16348, #17636, #2322, #7713, #1036 ) ) ;
#17943=CARTESIAN_POINT ( 'NONE',  ( 51.61786746416480298, 93.13668562621728597, 1.065498654441493720 ) ) ;
#17947=CARTESIAN_POINT ( 'NONE',  ( 47.97830229121277057, 144.4087953931572201, 33.55020052675504871 ) ) ;
#17953=CARTESIAN_POINT ( 'NONE',  ( 43.10205244623161036, 154.1398065127551149, -10.16071067355346358 ) ) ;
#17962=CARTESIAN_POINT ( 'NONE',  ( 22.02512380705847406, 92.75866610308527527, 21.07306443996510481 ) ) ;
#17966=CARTESIAN_POINT ( 'NONE',  ( 76.77449255912956971, 125.0547954796211485, -7.584917068115353267 ) ) ;
#17975=CARTESIAN_POINT ( 'NONE',  ( 73.72238702602700755, 135.0318370961144296, 5.077453337991364002 ) ) ;
#17985=CARTESIAN_POINT ( 'NONE',  ( 11.39584491653312526, 106.7788786240791978, 8.648593811254444930 ) ) ;
#17993=SURFACE_SIDE_STYLE ('',( #11273 ) ) ;
#18012=CARTESIAN_POINT ( 'NONE',  ( 14.73996261871784341, 120.6514404024884755, 15.19984638209844441 ) ) ;
#18018=CARTESIAN_POINT ( 'NONE',  ( 73.72238702602700755, 135.0318370961144296, 5.077453337991364002 ) ) ;
#18020=CARTESIAN_POINT ( 'NONE',  ( 70.22564533444385404, 112.8265553529472953, -14.05338489394683243 ) ) ;
#18025=ORIENTED_EDGE ( 'NONE', *, *, #8065, .T. ) ;
#18038=CARTESIAN_POINT ( 'NONE',  ( 35.88495058779732716, 86.34054347403214535, 13.57279861601404036 ) ) ;
#18044=CARTESIAN_POINT ( 'NONE',  ( 51.94691807752363388, 146.6530262932614050, -9.724486432582017059 ) ) ;
#18053=CARTESIAN_POINT ( 'NONE',  ( 36.14055301128134801, 147.1744539460121075, 4.637215583376333328 ) ) ;
#18065=CARTESIAN_POINT ( 'NONE',  ( 77.19215121279506775, 118.0176990621192203, -1.351406188750652992 ) ) ;
#18072=CARTESIAN_POINT ( 'NONE',  ( 68.49994877969884044, 96.93213776073638144, 19.40600457995573080 ) ) ;
#18075=CARTESIAN_POINT ( 'NONE',  ( 30.47730968207189051, 151.6776658675815384, -2.585197649422186661 ) ) ;
#18080=CARTESIAN_POINT ( 'NONE',  ( 71.07552608251525328, 117.1481954606975791, 12.77539325861266484 ) ) ;
#18085=CARTESIAN_POINT ( 'NONE',  ( 49.55020742284296631, 92.47612394764220767, 0.1565338505643876776 ) ) ;
#18097=CARTESIAN_POINT ( 'NONE',  ( 20.88913110926514705, 146.0313881486468119, 3.053432864643822686 ) ) ;
#18121=CARTESIAN_POINT ( 'NONE',  ( 14.82355424275916000, 117.6079223783217458, 15.08068057431173870 ) ) ;
#18127=DIRECTION ( 'NONE',  ( -0.000000000000000000, 1.000000000000000000, -0.000000000000000000 ) ) ;
#18128=CARTESIAN_POINT ( 'NONE',  ( 72.33162239183086228, 137.5781058455011703, 11.98183203572534872 ) ) ;
#18129=CARTESIAN_POINT ( 'NONE',  ( 37.89917375590665927, 147.5588116854153498, -9.291614562240097186 ) ) ;
#18148=CARTESIAN_POINT ( 'NONE',  ( 45.08439497331802670, 154.1588294112744677, 16.90626985941621641 ) ) ;
#18155=CARTESIAN_POINT ( 'NONE',  ( 17.64326796073342862, 132.3496329740814303, 22.67862939001841127 ) ) ;
#18165=CARTESIAN_POINT ( 'NONE',  ( 65.51498131554875215, 136.7693945797108199, 5.946615082358765569 ) ) ;
#18179=CARTESIAN_POINT ( 'NONE',  ( 50.92548328124963319, 86.60151408976496157, 0.07716523989554470442 ) ) ;
#18186=CARTESIAN_POINT ( 'NONE',  ( 9.116869730174032682, 125.2576736736073428, 22.26325814793822744 ) ) ;
#18189=CARTESIAN_POINT ( 'NONE',  ( 11.65896226128411683, 106.3627486108568547, -4.370744638174604013 ) ) ;
#18193=CARTESIAN_POINT ( 'NONE',  ( 27.67177345608778793, 143.5689829720894011, 10.27550654291302479 ) ) ;
#18199=CARTESIAN_POINT ( 'NONE',  ( 62.17156016504299032, 99.21662021101468554, 6.584824431686855384 ) ) ;
#18201=CARTESIAN_POINT ( 'NONE',  ( 28.07864021081662287, 89.10199518432737875, 14.83897397183228861 ) ) ;
#18213=CARTESIAN_POINT ( 'NONE',  ( 13.33420504782278293, 102.8437529505761603, 1.505736668420971869 ) ) ;
#18219=CARTESIAN_POINT ( 'NONE',  ( 15.75986397150585816, 99.18880659646561071, -5.637120474378671808 ) ) ;
#18220=VECTOR ( 'NONE', #15487, 1000.000000000000000 ) ;
#18241=CARTESIAN_POINT ( 'NONE',  ( 40.03295031927941494, 147.9482203214073479, -10.20071078494585670 ) ) ;
#18248=CARTESIAN_POINT ( 'NONE',  ( 11.39584491653312526, 106.7788786240791978, 8.648593811254444930 ) ) ;
#18250=CARTESIAN_POINT ( 'NONE',  ( 71.12409474721032154, 120.5409021055102841, -0.3630727742139398528 ) ) ;
#18266=CARTESIAN_POINT ( 'NONE',  ( 77.32109437525961937, 120.4276527761501399, 18.57288864564252506 ) ) ;
#18271=CARTESIAN_POINT ( 'NONE',  ( 11.38715737009742668, 107.0096734253407362, 2.652989958896663225 ) ) ;
#18273=CARTESIAN_POINT ( 'NONE',  ( 70.84063976188440392, 115.3547488198113200, -1.153064885589385025 ) ) ;
#18275=AXIS2_PLACEMENT_3D ( 'NONE', #3411, #1751, #18824 ) ;
#18285=CARTESIAN_POINT ( 'NONE',  ( 67.53959295026429288, 106.1551078129065075, 0.2323293680688409690 ) ) ;
#18296=CARTESIAN_POINT ( 'NONE',  ( 61.01612483116806374, 90.79174121657607088, -0.2798613066081144796 ) ) ;
#18303=CARTESIAN_POINT ( 'NONE',  ( 35.88495058779732716, 86.34054347403214535, 13.57279861601404036 ) ) ;
#18305=CARTESIAN_POINT ( 'NONE',  ( 76.02541712503827398, 128.6535784478189726, -7.704039830276845358 ) ) ;
#18316=CARTESIAN_POINT ( 'NONE',  ( 14.82803154953497859, 120.8649872489531987, 9.204245268424362081 ) ) ;
#18329=CARTESIAN_POINT ( 'NONE',  ( 46.60148787037231699, 85.86292235506145687, 7.220022382731924537 ) ) ;
#18335=CARTESIAN_POINT ( 'NONE',  ( 11.74529739132928619, 133.8467647624810581, -4.446451035385589279 ) ) ;
#18337=CARTESIAN_POINT ( 'NONE',  ( 70.05982654948900290, 127.8813624167294023, -8.653178033719973072 ) ) ;
#18343=CARTESIAN_POINT ( 'NONE',  ( 30.38027039762175718, 151.3010018550503446, 11.44158087452429129 ) ) ;
#18352=CARTESIAN_POINT ( 'NONE',  ( 61.21858502650649569, 141.5469622553929128, 17.69968404581608823 ) ) ;
#18359=CARTESIAN_POINT ( 'NONE',  ( 54.44380493464903736, 94.21656919670213881, 0.9465279732350617703 ) ) ;
#18378=CARTESIAN_POINT ( 'NONE',  ( 57.37541587618559191, 88.74458412249896355, 12.85860293144399513 ) ) ;
#18385=CARTESIAN_POINT ( 'NONE',  ( 41.83190538388809188, 154.0406478741334126, 4.796127949319595629 ) ) ;
#18386=CARTESIAN_POINT ( 'NONE',  ( 47.24326884731692644, 147.7868190896643341, 4.084992211255583427 ) ) ;
#18398=CARTESIAN_POINT ( 'NONE',  ( 25.43708531585104993, 141.8584285267105827, 4.160929998272084873 ) ) ;
#18409=CARTESIAN_POINT ( 'NONE',  ( 74.85601106972485752, 107.3429126181175661, -0.9942341299615756745 ) ) ;
#18419=CARTESIAN_POINT ( 'NONE',  ( 29.98029990418277180, 151.1550010424932111, 23.43402463578956585 ) ) ;
#18429=CARTESIAN_POINT ( 'NONE',  ( 29.72792815944318789, 144.7825833525567134, 3.370790685444458479 ) ) ;
#18431=CARTESIAN_POINT ( 'NONE',  ( 31.47436479266152531, 87.67613096727390598, 14.72005176623422606 ) ) ;
#18435=CARTESIAN_POINT ( 'NONE',  ( 38.26681966641773158, 144.4530603969024014, 32.59926919370181508 ) ) ;
#18441=CARTESIAN_POINT ( 'NONE',  ( 63.43270131736515083, 147.4839633491013728, -3.451138109367889228 ) ) ;
#18448=CARTESIAN_POINT ( 'NONE',  ( 32.31036143884366396, 152.4250368413922274, -10.51794503956956817 ) ) ;
#18450=CARTESIAN_POINT ( 'NONE',  ( 18.86999673272213229, 105.3337293714367604, -5.438779171309367833 ) ) ;
#18455=CARTESIAN_POINT ( 'NONE',  ( 77.22348061889915982, 118.7203125366680752, -8.375138532479306619 ) ) ;
#18464=CARTESIAN_POINT ( 'NONE',  ( 62.59245796673033624, 99.61375035622579333, -0.4388640268946644718 ) ) ;
#18471=CARTESIAN_POINT ( 'NONE',  ( 75.40436159597490473, 130.9804297329818326, 12.22031048084446248 ) ) ;
#18472=CARTESIAN_POINT ( 'NONE',  ( 14.91610048035210312, 121.0785340954179645, 3.208644154750278865 ) ) ;
#18487=CARTESIAN_POINT ( 'NONE',  ( 61.62447910614003632, 148.7338836329059859, 10.47761036752830144 ) ) ;
#18492=EDGE_CURVE ( 'NONE', #18531, #4997, #12201, .T. ) ;
#18493=CARTESIAN_POINT ( 'NONE',  ( 56.91482361236938203, 88.71218622616480332, 0.8673887411229855848 ) ) ;
#18494=CARTESIAN_POINT ( 'NONE',  ( 62.59245796673033624, 99.61375035622579333, -0.4388640268946644718 ) ) ;
#18505=CARTESIAN_POINT ( 'NONE',  ( 26.51748177580332566, 149.8140053266110385, -9.728054792207391444 ) ) ;
#18516=CARTESIAN_POINT ( 'NONE',  ( 69.83118287335672392, 141.1824132108841638, 4.838974892866481525 ) ) ;
#18524=CARTESIAN_POINT ( 'NONE',  ( 33.94330515458147346, 146.6952251797808628, -4.443226218224292978 ) ) ;
#18531=VERTEX_POINT ( 'NONE', #16767 ) ;
#18536=CARTESIAN_POINT ( 'NONE',  ( 20.72232308940363765, 137.1362251821529696, 16.90007324815861267 ) ) ;
#18551=CARTESIAN_POINT ( 'NONE',  ( 69.91774837562090283, 98.61087038541865013, -1.665158713316885919 ) ) ;
#18558=CARTESIAN_POINT ( 'NONE',  ( 8.927628897234525240, 116.7075971571176751, 1.981832035706394546 ) ) ;
#18560=CARTESIAN_POINT ( 'NONE',  ( 24.69269415895541542, 98.46806607146707790, -5.796035312751787849 ) ) ;
#18565=CARTESIAN_POINT ( 'NONE',  ( 77.16427934405430733, 119.9933672671919851, 6.581674455321548933 ) ) ;
#18574=CARTESIAN_POINT ( 'NONE',  ( 53.00431643774457768, 93.53749527547704190, -6.986323292181506162 ) ) ;
#18579=ORIENTED_EDGE ( 'NONE', *, *, #19622, .F. ) ;
#18581=CARTESIAN_POINT ( 'NONE',  ( 59.73150498404358899, 90.03452709159309109, 13.76780503130795097 ) ) ;
#18583=CARTESIAN_POINT ( 'NONE',  ( 25.97839122281734703, 97.53232036182296838, 2.136956866322798021 ) ) ;
#18588=EDGE_CURVE ( 'NONE', #4997, #19976, #3550, .T. ) ;
#18601=CARTESIAN_POINT ( 'NONE',  ( 41.36127970224624306, 91.67401929561202678, -0.5144393322287174053 ) ) ;
#18606=CARTESIAN_POINT ( 'NONE',  ( 22.17150742865759483, 138.9041494244890771, -4.010207742755246052 ) ) ;
#18615=CARTESIAN_POINT ( 'NONE',  ( 23.54274795406405474, 91.84646939011692268, -11.98975411606233976 ) ) ;
#18625=CARTESIAN_POINT ( 'NONE',  ( 65.27013532398795803, 145.9152199903044504, 11.62486143609835310 ) ) ;
#18632=CARTESIAN_POINT ( 'NONE',  ( 46.46425003030392986, 147.9761360841216344, 3.056716434341200106 ) ) ;
#18645=CARTESIAN_POINT ( 'NONE',  ( 69.05514009256096131, 130.5101840208823205, -14.76775785107876082 ) ) ;
#18656=CARTESIAN_POINT ( 'NONE',  ( 70.62757080055673953, 99.67629488849819097, 13.29148015538516425 ) ) ;
#18664=CARTESIAN_POINT ( 'NONE',  ( 36.38086904327614235, 86.32171732562966326, 0.5532606071062302622 ) ) ;
#18666=CARTESIAN_POINT ( 'NONE',  ( 58.35211712195835076, 96.24552883246097679, -7.224606741634919338 ) ) ;
#18673=CARTESIAN_POINT ( 'NONE',  ( 76.97600836722278927, 116.3222765712875031, 6.700797217583226661 ) ) ;
#18682=CARTESIAN_POINT ( 'NONE',  ( 20.57499262110235350, 102.8243204193801432, -5.557751863727047770 ) ) ;
#18692=CARTESIAN_POINT ( 'NONE',  ( 22.77429378292968920, 139.4308542021594519, -2.981927144630473148 ) ) ;
#18707=CARTESIAN_POINT ( 'NONE',  ( 69.60802376816022274, 110.2920722108499518, -1.943010761821444943 ) ) ;
#18711=CARTESIAN_POINT ( 'NONE',  ( 34.64294707643933435, 153.0196542278736729, 4.557659493426334585 ) ) ;
#18712=CARTESIAN_POINT ( 'NONE',  ( 24.69269415895541542, 98.46806607146707790, -5.796035312751787849 ) ) ;
#18715=VERTEX_POINT ( 'NONE', #10815 ) ;
#18721=CARTESIAN_POINT ( 'NONE',  ( 11.90670198672629354, 134.0117795012786814, -10.44205992529839122 ) ) ;
#18725=CARTESIAN_POINT ( 'NONE',  ( 20.98687704487253569, 141.7792436784441747, -11.00219731500033049 ) ) ;
#18733=CARTESIAN_POINT ( 'NONE',  ( 50.13766412853455279, 153.4730781396112889, -3.927228689826556707 ) ) ;
#18739=CARTESIAN_POINT ( 'NONE',  ( 10.92950091243491251, 131.9893946842779542, 22.49106082041198107 ) ) ;
#18751=CARTESIAN_POINT ( 'NONE',  ( 64.82873087846098770, 102.1656695083886603, -13.57732884656604355 ) ) ;
#18759=PRODUCT_DEFINITION_CONTEXT ( 'detailed design', #10848, 'design' ) ;
#18764=CARTESIAN_POINT ( 'NONE',  ( 30.18028515090226449, 151.2280014487717779, 17.43780275515692679 ) ) ;
#18770=CARTESIAN_POINT ( 'NONE',  ( 26.13368487350976110, 90.12329638092472806, 0.9106621812756837686 ) ) ;
#18772=CARTESIAN_POINT ( 'NONE',  ( 32.38101408406643600, 93.78751416920769657, -6.153149741203968404 ) ) ;
#18778=CARTESIAN_POINT ( 'NONE',  ( 73.40451243997107156, 135.6611253642151098, -1.946480675884423084 ) ) ;
#18781=UNCERTAINTY_MEASURE_WITH_UNIT (LENGTH_MEASURE( 1.000000000000000082E-05 ), #10190, 'distance_accuracy_value', 'NONE');
#18786=CARTESIAN_POINT ( 'NONE',  ( 35.25059181783574758, 92.79662968204097240, -6.272318425388238694 ) ) ;
#18795=CARTESIAN_POINT ( 'NONE',  ( 45.08035905667198762, 147.9511986603014861, 4.994099723559113357 ) ) ;
#18812=CARTESIAN_POINT ( 'NONE',  ( 53.23527110998836775, 93.53878102080766155, -0.9907194398206048414 ) ) ;
#18816=CARTESIAN_POINT ( 'NONE',  ( 18.86674891209846905, 143.9013856721611546, -11.04182128657428485 ) ) ;
#18817=CARTESIAN_POINT ( 'NONE',  ( 48.35156950851215640, 92.21792820573091376, 14.20396468032920012 ) ) ;
#18824=DIRECTION ( 'NONE',  ( 1.000000000000000000, 0.000000000000000000, -0.000000000000000000 ) ) ;
#18828=CARTESIAN_POINT ( 'NONE',  ( 43.31828379119179573, 154.0590585871367750, -16.15632009132952973 ) ) ;
#18838=CARTESIAN_POINT ( 'NONE',  ( 21.43032318156618388, 146.4805633285969861, 10.07716523980869816 ) ) ;
#18843=CARTESIAN_POINT ( 'NONE',  ( 58.57740969237692497, 96.29577388269515836, -1.228997851713355072 ) ) ;
#18854=CARTESIAN_POINT ( 'NONE',  ( 40.94005093944240059, 91.86375568685591020, -12.50564155961141566 ) ) ;
#18860=CARTESIAN_POINT ( 'NONE',  ( 47.97879638358897836, 95.40545967527941684, 33.55330648861601617 ) ) ;
#18867=CARTESIAN_POINT ( 'NONE',  ( 62.84376099716368458, 92.00366499689042143, 13.64888190966157566 ) ) ;
#18873=CARTESIAN_POINT ( 'NONE',  ( 14.15704070161504369, 138.3271338521546454, 9.720138693322796897 ) ) ;
#18875=CARTESIAN_POINT ( 'NONE',  ( 34.07414013685151843, 93.16113583794900421, 7.775673839875955728 ) ) ;
#18882=CARTESIAN_POINT ( 'NONE',  ( 74.85601106972485752, 107.3429126181175661, -0.9942341299615756745 ) ) ;
#18895=PRODUCT_DEFINITION ( 'UNKNOWN', '', #9864, #18759 ) ;
#18901=CARTESIAN_POINT ( 'NONE',  ( 59.05508021657500706, 143.0007772151335814, 5.589501426708507026 ) ) ;
#18922=CARTESIAN_POINT ( 'NONE',  ( 20.64193819951031017, 102.6032774297415102, 0.4378519886423143381 ) ) ;
#18929=CARTESIAN_POINT ( 'NONE',  ( 42.00398509169406935, 85.76881261499585207, 8.367275628961508005 ) ) ;
#18931=CARTESIAN_POINT ( 'NONE',  ( 39.35338560254503903, 91.94623120232463975, 14.56122079753911081 ) ) ;
#18941=CARTESIAN_POINT ( 'NONE',  ( 22.73392375623628681, 139.3438357627746882, 11.01889030017397531 ) ) ;
#18950=CARTESIAN_POINT ( 'NONE',  ( 59.73150498404358899, 90.03452709159309109, 13.76780503130795097 ) ) ;
#18956=CARTESIAN_POINT ( 'NONE',  ( 24.36338960932843634, 98.64599907776933208, 7.223456449276175029 ) ) ;
#18967=CARTESIAN_POINT ( 'NONE',  ( 17.98614708603287937, 106.9092867359673704, 15.63253669370310384 ) ) ;
#18972=CARTESIAN_POINT ( 'NONE',  ( 43.66822579977166896, 94.91365412844299954, 39.17808643222355869 ) ) ;
#18979=CARTESIAN_POINT ( 'NONE',  ( 8.701189160817120793, 119.3880529461122109, 1.073064441167490557 ) ) ;
#18985=CARTESIAN_POINT ( 'NONE',  ( 76.66991938639012005, 113.6622739410785670, 5.791450954060403333 ) ) ;
#18988=CARTESIAN_POINT ( 'NONE',  ( 37.56771007382699423, 92.23784766911828115, 0.6328166970475824771 ) ) ;
#18998=CARTESIAN_POINT ( 'NONE',  ( 9.656473946750173454, 127.6128973189080398, 2.339233609801092406 ) ) ;
#19009=DIRECTION ( 'NONE',  ( -0.000000000000000000, 1.000000000000000000, -0.000000000000000000 ) ) ;
#19014=CARTESIAN_POINT ( 'NONE',  ( 70.97434162403952485, 116.9407273601718202, 6.779784368693626995 ) ) ;
#19020=( GEOMETRIC_REPRESENTATION_CONTEXT ( 3 ) GLOBAL_UNCERTAINTY_ASSIGNED_CONTEXT ( ( #20761 ) ) GLOBAL_UNIT_ASSIGNED_CONTEXT ( ( #14733, #2830, #17706 ) ) REPRESENTATION_CONTEXT ( 'NONE', 'WORKASPACE' ) );
#19032=CARTESIAN_POINT ( 'NONE',  ( 24.57236314005146838, 141.2733614120550385, -4.872173989822636386 ) ) ;
#19039=CARTESIAN_POINT ( 'NONE',  ( 17.73005198514846725, 142.9879744078657779, -4.089424278207452801 ) ) ;
#19041=CARTESIAN_POINT ( 'NONE',  ( 14.82803154953497859, 120.8649872489531987, 9.204245268424362081 ) ) ;
#19049=CARTESIAN_POINT ( 'NONE',  ( 53.48172298457406271, 87.39834721931525507, 0.9865115032505324955 ) ) ;
#19058=CARTESIAN_POINT ( 'NONE',  ( 28.07864021081662287, 89.10199518432737875, 14.83897397183228861 ) ) ;
#19064=EDGE_CURVE ( 'NONE', #5848, #21236, #14864, .T. ) ;
#19065=CARTESIAN_POINT ( 'NONE',  ( 20.79828168028384994, 137.4105449198869735, 15.91385929137521771 ) ) ;
#19076=CARTESIAN_POINT ( 'NONE',  ( 15.11514590861459162, 123.4468881749472615, -3.696500957071167104 ) ) ;
#19089=ORIENTED_EDGE ( 'NONE', *, *, #11081, .F. ) ;
#19091=CARTESIAN_POINT ( 'NONE',  ( 36.57762280775352082, 86.20069522707665044, 6.548861720777491513 ) ) ;
#19101=CARTESIAN_POINT ( 'NONE',  ( 55.81398226145393693, 145.0329042473489096, 4.442248136324586483 ) ) ;
#19107=CARTESIAN_POINT ( 'NONE',  ( 30.08091612619420729, 88.20954595054467973, -6.232194961517499188 ) ) ;
#19111=CARTESIAN_POINT ( 'NONE',  ( 43.01140435219951996, 119.9070776186055838, -19.99999999999997868 ) ) ;
#19118=CARTESIAN_POINT ( 'NONE',  ( 55.11952973528949684, 87.88698225678692211, -7.065691903092018222 ) ) ;
#19125=CARTESIAN_POINT ( 'NONE',  ( 17.95776995827587896, 107.1383635228311846, 9.636927859708212196 ) ) ;
#19139=CARTESIAN_POINT ( 'NONE',  ( 66.44170838958859804, 135.7440291252205213, 4.009006963233090026 ) ) ;
#19144=CARTESIAN_POINT ( 'NONE',  ( 14.43535904578935103, 101.2031681353820574, 9.438814132600386486 ) ) ;
#19145=CARTESIAN_POINT ( 'NONE',  ( 37.00104444766353851, 92.35499785847434850, 7.656504971210453370 ) ) ;
#19153=CARTESIAN_POINT ( 'NONE',  ( 17.06177112331949886, 97.70250936324737268, 2.295960169688653352 ) ) ;
#19155=CARTESIAN_POINT ( 'NONE',  ( 28.07864021081662287, 89.10199518432737875, 14.83897397183228861 ) ) ;
#19162=CARTESIAN_POINT ( 'NONE',  ( 69.91774837562090283, 98.61087038541865013, -1.665158713316885919 ) ) ;
#19169=CARTESIAN_POINT ( 'NONE',  ( 17.21810733192966936, 108.3100148859214329, 7.699684045823485867 ) ) ;
#19172=VERTEX_POINT ( 'NONE', #14971 ) ;
#19181=CARTESIAN_POINT ( 'NONE',  ( 66.54750331441660194, 135.2948500229566093, -7.982215242636039321 ) ) ;
#19196=CARTESIAN_POINT ( 'NONE',  ( 69.75981547520746062, 141.4021063757441823, 10.83457600654633879 ) ) ;
#19203=CARTESIAN_POINT ( 'NONE',  ( 70.21798013780751546, 127.3226622636268672, -1.629293503064584536 ) ) ;
#19210=CARTESIAN_POINT ( 'NONE',  ( 16.30372524420941716, 141.3216567370616019, 9.839263250375132941 ) ) ;
#19220=CARTESIAN_POINT ( 'NONE',  ( 68.88151390383544026, 142.3271613368909811, -9.208263745312144977 ) ) ;
#19227=CARTESIAN_POINT ( 'NONE',  ( 30.56769828357572294, 94.69056354510921381, 8.922930725513751327 ) ) ;
#19245=CARTESIAN_POINT ( 'NONE',  ( 60.26010703883354580, 142.3196469542212697, 3.652109145728902551 ) ) ;
#19250=CARTESIAN_POINT ( 'NONE',  ( 67.39040179371399120, 143.9404232637865562, 4.720051584306741432 ) ) ;
#19252=CARTESIAN_POINT ( 'NONE',  ( 27.67177345608778793, 143.5689829720894011, 10.27550654291302479 ) ) ;
#19262=CARTESIAN_POINT ( 'NONE',  ( 50.69626032627856915, 86.62977272806217854, -5.918438612465169335 ) ) ;
#19266=CARTESIAN_POINT ( 'NONE',  ( 77.07719282571002850, 116.5297446719512209, 12.69640610750513865 ) ) ;
#19271=CARTESIAN_POINT ( 'NONE',  ( 72.04953363923264931, 101.6246461802091972, -1.784078408812360017 ) ) ;
#19277=CARTESIAN_POINT ( 'NONE',  ( 14.90453237821946253, 123.0362832886413855, 8.294721248935834623 ) ) ;
#19289=CARTESIAN_POINT ( 'NONE',  ( 17.19109055900979399, 108.7710072034773532, -4.291528102762561581 ) ) ;
#19297=CARTESIAN_POINT ( 'NONE',  ( 23.23160898551418185, 147.7622765488190453, -10.85157364460736140 ) ) ;
#19301=EDGE_LOOP ( 'NONE', ( #15607, #12823 ) ) ;
#19302=CARTESIAN_POINT ( 'NONE',  ( 20.67200536010596323, 145.9528555770810385, 9.049038938933962939 ) ) ;
#19309=CARTESIAN_POINT ( 'NONE',  ( 49.55020742284296631, 92.47612394764220767, 0.1565338505643876776 ) ) ;
#19316=CARTESIAN_POINT ( 'NONE',  ( 41.61242760320212852, 154.1118385459532760, 10.79173905232880237 ) ) ;
#19325=CARTESIAN_POINT ( 'NONE',  ( 75.10802748102119608, 108.0013139708956800, -8.018167963582932600 ) ) ;
#19339=CARTESIAN_POINT ( 'NONE',  ( 33.01140435219951286, 119.9070776186055838, 8.284271247461942878 ) ) ;
#19349=CARTESIAN_POINT ( 'NONE',  ( 70.95506224315714405, 115.5552942049593668, 4.842541188697900623 ) ) ;
#19355=CARTESIAN_POINT ( 'NONE',  ( 58.57487293839693621, 150.3975950434478648, 4.362879525569486994 ) ) ;
#19356=CARTESIAN_POINT ( 'NONE',  ( 64.38652456388278722, 138.1782414180340197, -15.12506982898978158 ) ) ;
#19366=CARTESIAN_POINT ( 'NONE',  ( 74.70172802024292480, 107.1710682803345662, -6.989838304517381751 ) ) ;
#19376=CARTESIAN_POINT ( 'NONE',  ( 17.69433683334896656, 96.74512228834443306, 7.263443568815639573 ) ) ;
#19381=CARTESIAN_POINT ( 'NONE',  ( 40.78231060393920870, 91.71360054188218669, 6.509252002934985626 ) ) ;
#19391=CARTESIAN_POINT ( 'NONE',  ( 14.89151287784495281, 119.8505320279099209, -10.83935810001172229 ) ) ;
#19393=CARTESIAN_POINT ( 'NONE',  ( 46.31959713345366225, 144.6883137394385130, 37.97384977752898294 ) ) ;
#19405=CARTESIAN_POINT ( 'NONE',  ( 58.41865009756546812, 150.5677012977470781, 10.35848337793017393 ) ) ;
#19412=CARTESIAN_POINT ( 'NONE',  ( 25.21830160582964453, 141.7844325674071229, 10.15653385063274428 ) ) ;
#19420=CARTESIAN_POINT ( 'NONE',  ( 59.73150498404358899, 90.03452709159309109, 13.76780503130795097 ) ) ;
#19421=CARTESIAN_POINT ( 'NONE',  ( 42.35335639509444405, 94.91365384002462235, 39.17809732472422724 ) ) ;
#19426=AXIS2_PLACEMENT_3D ( 'NONE', #5209, #20102, #4991 ) ;
#19432=CARTESIAN_POINT ( 'NONE',  ( 11.74529739132928619, 133.8467647624810581, -4.446451035385589279 ) ) ;
#19435=ORIENTED_EDGE ( 'NONE', *, *, #21507, .T. ) ;
#19457=CARTESIAN_POINT ( 'NONE',  ( 70.86003890729777766, 114.9808142912368254, 11.86642341732858874 ) ) ;
#19463=CARTESIAN_POINT ( 'NONE',  ( 35.69068542950036260, 86.46542255174357194, 7.577194441455407770 ) ) ;
#19464=CARTESIAN_POINT ( 'NONE',  ( 43.96673757894181023, 91.80305570246190427, -12.62481348914368873 ) ) ;
#19465=CARTESIAN_POINT ( 'NONE',  ( 55.11952973528949684, 87.88698225678692211, -7.065691903092018222 ) ) ;
#19473=CARTESIAN_POINT ( 'NONE',  ( 13.29607544193514990, 103.0715419909171970, -4.489867183945484896 ) ) ;
#19475=CARTESIAN_POINT ( 'NONE',  ( 34.41316853928974950, 153.0433231119815503, 10.55326060710041958 ) ) ;
#19481=CARTESIAN_POINT ( 'NONE',  ( 77.21761637129371536, 122.6259224659223861, -2.498659462202352799 ) ) ;
#19483=CARTESIAN_POINT ( 'NONE',  ( 185.6125732647967368, 204.7716666330005921, 23.27362312593913174 ) ) ;
#19485=CARTESIAN_POINT ( 'NONE',  ( 43.01140435219951996, 119.9070776186055838, -19.99999999999998579 ) ) ;
#19487=CARTESIAN_POINT ( 'NONE',  ( 18.01452421378985136, 106.6802099491036273, 21.62814552769798837 ) ) ;
#19498=CARTESIAN_POINT ( 'NONE',  ( 40.36503175183082703, 91.91162403226272204, -5.481956346182379924 ) ) ;
#19500=CARTESIAN_POINT ( 'NONE',  ( 47.75437220321179410, 144.4533750968706158, 32.59446367923829513 ) ) ;
#19505=CARTESIAN_POINT ( 'NONE',  ( 60.49690154327523572, 149.3382625450468311, -9.565656633516235630 ) ) ;
#19506=VECTOR ( 'NONE', #10276, 1000.000000000000000 ) ;
#19513=CARTESIAN_POINT ( 'NONE',  ( 70.19659433329162823, 140.8466096914638399, 17.85851290171837746 ) ) ;
#19523=AXIS2_PLACEMENT_3D ( 'NONE', #9248, #21038, #5921 ) ;
#19528=CARTESIAN_POINT ( 'NONE',  ( 40.36769960724004846, 95.04687716051704172, 29.96360841760569471 ) ) ;
#19535=CARTESIAN_POINT ( 'NONE',  ( 13.69124840528610321, 102.2378096837820181, -5.517995706778950016 ) ) ;
#19559=CARTESIAN_POINT ( 'NONE',  ( 69.49514557983670215, 129.8286863358667347, 11.27102936561352742 ) ) ;
#19567=CARTESIAN_POINT ( 'NONE',  ( 29.43094928344231320, 88.48265962617873015, 0.7917390523231137012 ) ) ;
#19568=CARTESIAN_POINT ( 'NONE',  ( 62.76710561173204894, 139.9178416638646638, -8.219927273936241008 ) ) ;
#19579=CARTESIAN_POINT ( 'NONE',  ( 23.63511980923729183, 148.0372221624750466, 11.16864677238829984 ) ) ;
#19588=CARTESIAN_POINT ( 'NONE',  ( 26.06094713673110164, 149.7432261477326563, 2.263147435255992601 ) ) ;
#19590=FACE_OUTER_BOUND ( 'NONE', #19301, .T. ) ;
#19596=CARTESIAN_POINT ( 'NONE',  ( 29.27949416537561333, 144.5119445999418986, 23.32977622066093204 ) ) ;
#19599=EDGE_CURVE ( 'NONE', #17523, #12901, #10996, .T. ) ;
#19608=CARTESIAN_POINT ( 'NONE',  ( 16.96697132366095673, 109.3049078165896901, 2.732358569689224748 ) ) ;
#19610=CARTESIAN_POINT ( 'NONE',  ( 47.85221094865248403, 144.4340178052514716, 35.50423386912935086 ) ) ;
#19616=CARTESIAN_POINT ( 'NONE',  ( 50.33192209904863290, 153.3481575868430014, -9.922832680162505525 ) ) ;
#19622=EDGE_CURVE ( 'NONE', #18715, #5848, #17752, .T. ) ;
#19626=CARTESIAN_POINT ( 'NONE',  ( 57.37541587618559191, 88.74458412249896355, 12.85860293144399513 ) ) ;
#19630=CARTESIAN_POINT ( 'NONE',  ( 36.78388215320455856, 153.4884242111695301, -9.370659782632428048 ) ) ;
#19643=CARTESIAN_POINT ( 'NONE',  ( 8.869018199820361659, 117.4101421016551967, 9.005765870029716069 ) ) ;
#19644=CARTESIAN_POINT ( 'NONE',  ( 39.70321157094539188, 95.12584149777269715, 37.97384977752899715 ) ) ;
#19653=CARTESIAN_POINT ( 'NONE',  ( 57.14511974427749408, 88.72838517433189054, 6.862995836283489304 ) ) ;
#19661=FILL_AREA_STYLE ('',( #12937 ) ) ;
#19677=CARTESIAN_POINT ( 'NONE',  ( 65.38103680468944390, 137.2114283014329317, 17.93782343147312730 ) ) ;
#19684=CARTESIAN_POINT ( 'NONE',  ( 51.78234217841457365, 152.9971814535558963, 4.124977536042813142 ) ) ;
#19685=CARTESIAN_POINT ( 'NONE',  ( 29.48178659935447854, 144.5857871963822845, 17.33364154221121467 ) ) ;
#19704=CARTESIAN_POINT ( 'NONE',  ( 22.58852954093744714, 92.33198060352846426, 14.04912700239559520 ) ) ;
#19710=CARTESIAN_POINT ( 'NONE',  ( 41.61464536962099459, 148.1530905165343768, 16.86614982034995691 ) ) ;
#19720=CARTESIAN_POINT ( 'NONE',  ( 70.89290225163276205, 123.5572941793614206, -0.4820434552990647825 ) ) ;
#19723=DIRECTION ( 'NONE',  ( -0.000000000000000000, -0.000000000000000000, -1.000000000000000000 ) ) ;
#19737=CARTESIAN_POINT ( 'NONE',  ( 16.10574266336056226, 141.2029798434031989, 15.83487214029357659 ) ) ;
#19741=CARTESIAN_POINT ( 'NONE',  ( 39.81857293680397447, 85.90283706545402254, -5.561266875997713299 ) ) ;
#19744=CARTESIAN_POINT ( 'NONE',  ( 50.77370750611731154, 147.0167679772302165, 11.22784935402935957 ) ) ;
#19752=CARTESIAN_POINT ( 'NONE',  ( 50.77370750611731154, 147.0167679772302165, 11.22784935402935957 ) ) ;
#19755=CARTESIAN_POINT ( 'NONE',  ( 40.50968990821500171, 95.03214066145851291, 29.87844397536261454 ) ) ;
#19758=CARTESIAN_POINT ( 'NONE',  ( 40.79112291011433200, 144.8101386900725061, 38.70263932541808316 ) ) ;
#19764=CARTESIAN_POINT ( 'NONE',  ( 16.30372524420941716, 141.3216567370616019, 9.839263250375132941 ) ) ;
#19780=CARTESIAN_POINT ( 'NONE',  ( 185.6125732647967368, 204.7716666330005921, 23.27362312593913174 ) ) ;
#19790=CARTESIAN_POINT ( 'NONE',  ( 71.17671054099098171, 117.3556635612232810, 18.77100214853170357 ) ) ;
#19795=DIRECTION ( 'NONE',  ( 0.000000000000000000, 0.000000000000000000, 1.000000000000000000 ) ) ;
#19796=CARTESIAN_POINT ( 'NONE',  ( 45.29500579500201951, 154.0643053174194961, 10.91066218119221709 ) ) ;
#19798=CARTESIAN_POINT ( 'NONE',  ( 20.44379504597808861, 136.6827000062168338, -10.12478428749056469 ) ) ;
#19799=AXIS2_PLACEMENT_3D ( 'NONE', #17719, #17615, #6372 ) ;
#19815=CARTESIAN_POINT ( 'NONE',  ( 34.18339000214019308, 153.0669919960894845, 16.54886172077450368 ) ) ;
#19821=CARTESIAN_POINT ( 'NONE',  ( 57.03263806925237844, 95.34629841206742640, 19.84245794357962822 ) ) ;
#19830=CARTESIAN_POINT ( 'NONE',  ( 33.89447768034496278, 93.30632465966320410, 1.780072726204736000 ) ) ;
#19841=CARTESIAN_POINT ( 'NONE',  ( 61.76154402333882132, 148.5480768402654803, 4.482004293238171400 ) ) ;
#19847=CARTESIAN_POINT ( 'NONE',  ( 46.82521527361338087, 85.80558333884177102, 13.21562623509259282 ) ) ;
#19851=CARTESIAN_POINT ( 'NONE',  ( 66.98923854426821833, 144.2286169274386509, -8.299483363615854259 ) ) ;
#19852=ORIENTED_EDGE ( 'NONE', *, *, #18492, .F. ) ;
#19856=CARTESIAN_POINT ( 'NONE',  ( 67.15412698936957270, 134.4792784496449087, 12.06138812558265805 ) ) ;
#19863=CARTESIAN_POINT ( 'NONE',  ( 46.56541826512206228, 91.93282113015048651, 0.2755065429245392439 ) ) ;
#19867=CARTESIAN_POINT ( 'NONE',  ( 23.42018083028975184, 147.9700754799198705, 17.16443675223517573 ) ) ;
#19876=CARTESIAN_POINT ( 'NONE',  ( 22.46358530849972723, 92.52609567587644790, 8.053519324161520387 ) ) ;
#19883=CARTESIAN_POINT ( 'NONE',  ( 13.69124840528610321, 102.2378096837820181, -5.517995706778950016 ) ) ;
#19903=CARTESIAN_POINT ( 'NONE',  ( 48.57925227495098852, 92.17995633088730756, 20.19957357060707182 ) ) ;
#19912=CARTESIAN_POINT ( 'NONE',  ( 14.99696000743431235, 117.4761687382565327, -3.934212988072375516 ) ) ;
#19928=CARTESIAN_POINT ( 'NONE',  ( 24.18607167610233333, 148.5957190367184353, 16.19189608183989648 ) ) ;
#19936=CARTESIAN_POINT ( 'NONE',  ( 63.19260820189420969, 92.35335041358771946, 0.6293402173502762320 ) ) ;
#19937=CARTESIAN_POINT ( 'NONE',  ( 34.17400395940548918, 146.6865494356538875, -10.43883331896520694 ) ) ;
#19940=VECTOR ( 'NONE', #6295, 1000.000000000000000 ) ;
#19949=CARTESIAN_POINT ( 'NONE',  ( 50.95956618318000864, 146.8798181090472212, 5.232242258870305918 ) ) ;
#19962=CARTESIAN_POINT ( 'NONE',  ( 76.81974253126139729, 125.2811442093199616, -1.589308178208348910 ) ) ;
#19970=CARTESIAN_POINT ( 'NONE',  ( 22.58852954093744714, 92.33198060352846426, 14.04912700239559520 ) ) ;
#19973=CARTESIAN_POINT ( 'NONE',  ( 44.19315180539718568, 85.77372119115894122, -12.70412401877768005 ) ) ;
#19976=VERTEX_POINT ( 'NONE', #12259 ) ;
#19982=CARTESIAN_POINT ( 'NONE',  ( 19.85370653151704090, 103.8158566922722486, 8.489678972899794118 ) ) ;
#19989=CARTESIAN_POINT ( 'NONE',  ( 38.01153310497667093, 144.4020013279858290, 34.53968432338326977 ) ) ;
#19990=PRODUCT ( 'Handle Balance Tension Spring', 'Handle Balance Tension Spring', '', ( #20897 ) ) ;
#19996=CARTESIAN_POINT ( 'NONE',  ( 9.656473946750173454, 127.6128973189080398, 2.339233609801092406 ) ) ;
#20002=CARTESIAN_POINT ( 'NONE',  ( 30.08091612619420729, 88.20954595054467973, -6.232194961517499188 ) ) ;
#20005=CARTESIAN_POINT ( 'NONE',  ( 20.57499262110235350, 102.8243204193801432, -5.557751863727047770 ) ) ;
#20012=CARTESIAN_POINT ( 'NONE',  ( 43.10205244623161036, 154.1398065127551149, -10.16071067355346358 ) ) ;
#20022=CARTESIAN_POINT ( 'NONE',  ( 59.59119729515064279, 96.99641097138604096, 19.72329267725583080 ) ) ;
#20029=LINE ( 'NONE', #5241, #18220 ) ;
#20030=CARTESIAN_POINT ( 'NONE',  ( 49.46632042442519861, 86.28835692931116341, 14.12497754236212977 ) ) ;
#20032=CARTESIAN_POINT ( 'NONE',  ( 37.37095630934955892, 92.35886976769425871, -5.362784416626555029 ) ) ;
#20049=CARTESIAN_POINT ( 'NONE',  ( 77.30322022806339533, 121.1324128411339984, 11.54915785461027511 ) ) ;
#20053=CARTESIAN_POINT ( 'NONE',  ( 22.33864107606189719, 92.72021074822440312, 2.057911645927444244 ) ) ;
#20054=CARTESIAN_POINT ( 'NONE',  ( 24.77189431714078083, 141.4131305960171687, 3.132649400142189844 ) ) ;
#20066=CARTESIAN_POINT ( 'NONE',  ( 69.68093098098093208, 128.8215514297462789, 6.303499042945750475 ) ) ;
#20076=CARTESIAN_POINT ( 'NONE',  ( 11.67247064774405452, 106.1322524520788875, 1.624861436118421043 ) ) ;
#20080=ORIENTED_EDGE ( 'NONE', *, *, #4507, .T. ) ;
#20083=CARTESIAN_POINT ( 'NONE',  ( 65.22477088018504787, 102.4029861919955948, -1.586113490162427864 ) ) ;
#20086=CARTESIAN_POINT ( 'NONE',  ( 33.21234449867455396, 152.6251194638087725, -9.489586336475131390 ) ) ;
#20094=CARTESIAN_POINT ( 'NONE',  ( 26.10333545525518062, 97.33820528946348816, 8.132564544556878161 ) ) ;
#20101=CARTESIAN_POINT ( 'NONE',  ( 38.68091485423948939, 144.5292836280306972, 31.70594869545380945 ) ) ;
#20102=DIRECTION ( 'NONE',  ( 0.9387810623359078566, 0.3426822732243069436, 0.03548206049944095664 ) ) ;
#20106=CARTESIAN_POINT ( 'NONE',  ( 23.42018083028975184, 147.9700754799198705, 17.16443675223517573 ) ) ;
#20114=CARTESIAN_POINT ( 'NONE',  ( 26.65597624659334031, 142.8797025615743337, -3.772066457372480475 ) ) ;
#20115=ORIENTED_EDGE ( 'NONE', *, *, #3491, .T. ) ;
#20120=CARTESIAN_POINT ( 'NONE',  ( 74.62708615766334219, 133.0342049366344384, -8.851289726714327344 ) ) ;
#20128=CARTESIAN_POINT ( 'NONE',  ( 15.06790588970514833, 124.2609462974868677, 22.34264618625151044 ) ) ;
#20134=CARTESIAN_POINT ( 'NONE',  ( 8.869018199820361659, 117.4101421016551967, 9.005765870029716069 ) ) ;
#20135=CARTESIAN_POINT ( 'NONE',  ( 62.38089001705685632, 99.52138843117178624, -6.434471705120163421 ) ) ;
#20153=CARTESIAN_POINT ( 'NONE',  ( 13.60337824163328513, 137.5875211305428252, 8.692014997358331385 ) ) ;
#20160=CARTESIAN_POINT ( 'NONE',  ( 72.81290617574171620, 103.2231620977376281, 0.1530188383368442095 ) ) ;
#20161=CARTESIAN_POINT ( 'NONE',  ( 50.11350838007777497, 92.61696660072725251, -6.867350599827054758 ) ) ;
#20173=CARTESIAN_POINT ( 'NONE',  ( 64.37283757718545019, 93.25908544850187809, -13.41832554473225692 ) ) ;
#20181=CARTESIAN_POINT ( 'NONE',  ( 66.24914683137549787, 94.76885710642066840, 6.506024766557033878 ) ) ;
#20188=CARTESIAN_POINT ( 'NONE',  ( 32.55111017628423298, 93.63144033427927582, -0.1575420629755377999 ) ) ;
#20198=CARTESIAN_POINT ( 'NONE',  ( 67.71458430423905384, 106.3058120325361671, 6.227933542621733487 ) ) ;
#20200=CARTESIAN_POINT ( 'NONE',  ( 9.203281625063985061, 114.5318647093721864, 15.91056058043385413 ) ) ;
#20204=CARTESIAN_POINT ( 'NONE',  ( 39.96131221638199804, 144.7218222453713565, 38.18604851697274682 ) ) ;
#20209=CARTESIAN_POINT ( 'NONE',  ( 68.80033453084351436, 142.5431462587704061, -3.212652714419679700 ) ) ;
#20214=DIRECTION ( 'NONE',  ( -1.186952418100008983E-16, -0.000000000000000000, -1.000000000000000000 ) ) ;
#20216=CARTESIAN_POINT ( 'NONE',  ( 51.60797029699607918, 86.77139250312444574, -6.946567135388369785 ) ) ;
#20218=CARTESIAN_POINT ( 'NONE',  ( 55.29376081731632553, 145.2908078538121401, -2.581636314160848489 ) ) ;
#20225=CARTESIAN_POINT ( 'NONE',  ( 74.11624783127615501, 105.8034190341144978, 7.057826790323951549 ) ) ;
#20234=CARTESIAN_POINT ( 'NONE',  ( 52.49585387951581339, 146.4637788833130685, -2.700609006624497876 ) ) ;
#20242=CARTESIAN_POINT ( 'NONE',  ( 17.14282613681034917, 97.48634091255654255, 8.291567264837656381 ) ) ;
#20244=CARTESIAN_POINT ( 'NONE',  ( 19.79626631456835284, 104.0394230781280669, 2.494070082984220171 ) ) ;
#20258=CARTESIAN_POINT ( 'NONE',  ( 44.40591325931411859, 91.66001841764941105, -0.6336051400208910778 ) ) ;
#20262=CARTESIAN_POINT ( 'NONE',  ( 58.73109577922829061, 150.2274887891485662, -1.632724326791204605 ) ) ;
#20264=CARTESIAN_POINT ( 'NONE',  ( 15.50679444821833819, 113.6848169819070193, -5.081469017220888063 ) ) ;
#20274=CARTESIAN_POINT ( 'NONE',  ( 77.08865571979157494, 122.1823731668103221, -14.48986716664726870 ) ) ;
#20283=CARTESIAN_POINT ( 'NONE',  ( 70.26356658872128946, 140.6255928306487704, 11.86290872716119615 ) ) ;
#20290=CARTESIAN_POINT ( 'NONE',  ( 51.76721073900363734, 146.7980033588722506, -3.728880589165500137 ) ) ;
#20294=CARTESIAN_POINT ( 'NONE',  ( 185.6125732647967368, 204.7716666330005921, 23.27362312593913174 ) ) ;
#20300=CARTESIAN_POINT ( 'NONE',  ( 57.54249972904700172, 143.9818934734506115, -15.48196187774845356 ) ) ;
#20315=CARTESIAN_POINT ( 'NONE',  ( 76.33227852969314142, 111.7084249013780806, -2.141487123205697340 ) ) ;
#20321=CARTESIAN_POINT ( 'NONE',  ( 57.78275410301085913, 89.02518083909171764, -0.1607367497116551913 ) ) ;
#20324=CARTESIAN_POINT ( 'NONE',  ( 69.04633063039527485, 130.7408809369782716, -8.772150750671475095 ) ) ;
#20331=CARTESIAN_POINT ( 'NONE',  ( 45.50561661668613311, 153.9697812235645245, 4.915054502968218664 ) ) ;
#20340=CARTESIAN_POINT ( 'NONE',  ( 29.22050282933603071, 144.5044581412665536, -3.652897588741476742 ) ) ;
#20349=CARTESIAN_POINT ( 'NONE',  ( 67.81612255856859406, 106.6615363072494915, -6.791355845220972576 ) ) ;
#20365=CARTESIAN_POINT ( 'NONE',  ( 59.79647059797250819, 142.6686746773435459, -3.371582063846674693 ) ) ;
#20369=CARTESIAN_POINT ( 'NONE',  ( 11.06625761453251933, 131.9899775861109106, 3.486483074593720755 ) ) ;
#20370=CARTESIAN_POINT ( 'NONE',  ( 71.16904767199986281, 118.3707548728134213, -1.272037577920760665 ) ) ;
#20380=CARTESIAN_POINT ( 'NONE',  ( 8.857566569312460558, 119.8222194325741725, -10.91815776494309098 ) ) ;
#20389=CARTESIAN_POINT ( 'NONE',  ( 53.04203944364535772, 87.17698241397053494, 14.00585298808814194 ) ) ;
#20396=CARTESIAN_POINT ( 'NONE',  ( 24.80496442426440140, 98.26638142913259344, 0.1995735771552373528 ) ) ;
#20397=SURFACE_STYLE_FILL_AREA ( #6956 ) ;
#20407=CARTESIAN_POINT ( 'NONE',  ( 30.72731853479779929, 94.52359049060457608, 14.91853181686295038 ) ) ;
#20413=CARTESIAN_POINT ( 'NONE',  ( 47.75426913703832099, 95.36076719471033414, 35.82660397859488199 ) ) ;
#20420=CARTESIAN_POINT ( 'NONE',  ( 70.26356658872128946, 140.6255928306487704, 11.86290872716119615 ) ) ;
#20427=CARTESIAN_POINT ( 'NONE',  ( 53.71239221804358976, 87.38980250447106357, 6.982120393166105998 ) ) ;
#20430=CARTESIAN_POINT ( 'NONE',  ( 24.78883071187807730, 141.3519591882296709, -10.86778418981948846 ) ) ;
#20436=CARTESIAN_POINT ( 'NONE',  ( 37.24990543953586553, 153.6521207556136517, 3.648881909465930828 ) ) ;
#20446=CARTESIAN_POINT ( 'NONE',  ( 22.17150742865759483, 138.9041494244890771, -4.010207742755246052 ) ) ;
#20455=CARTESIAN_POINT ( 'NONE',  ( 25.52315018325464635, 97.88680518890443238, 9.160641959101482712 ) ) ;
#20473=CARTESIAN_POINT ( 'NONE',  ( 21.96620680132455306, 138.7984961796735490, 1.985398331534963923 ) ) ;
#20477=CARTESIAN_POINT ( 'NONE',  ( 63.55746018358933469, 147.2895578332197033, -9.446739241148069510 ) ) ;
#20479=CARTESIAN_POINT ( 'NONE',  ( 70.51576897149806200, 126.1317638695992116, 12.41827883020830470 ) ) ;
#20480=ADVANCED_FACE ( 'NONE', ( #16728 ), #12092, .T. ) ;
#20490=CARTESIAN_POINT ( 'NONE',  ( 21.13084688720937976, 146.0403058103794649, -16.94226050084479596 ) ) ;
#20491=B_SPLINE_CURVE_WITH_KNOTS ( 'NONE', 3,
 ( #4425, #9628, #7971, #21418, #6307, #19758, #13472, #20204, #5312, #16983, #4990, #10390, #3335, #8735, #11700, #3554, #19989, #21642, #6977, #8627, #18435, #10063, #12023, #20101, #5097, #1792, #6656, #11814, #8523, #4875, #21747, #6865, #1891, #15345, #17090, #15237 ),
 .UNSPECIFIED., .F., .F.,
 ( 4, 2, 2, 2, 2, 2, 2, 2, 2, 2, 2, 2, 2, 2, 2, 2, 2, 4 ),
 ( 6.938893903907227607E-18, 0.0009794911224654358813, 0.001958982244930864824, 0.002938473367396293983, 0.003917964489861722709, 0.004897455612327151868, 0.005876946734792581027, 0.006856437857258010186, 0.007835928979723438478, 0.008815420102188867638, 0.009794911224654296797, 0.01028465678588701658, 0.01077440234711973810, 0.01175389346958516552, 0.01273338459205059121, 0.01371287571451601690, 0.01469236683698144086, 0.01567185795944686655 ),
 .UNSPECIFIED. ) ;
#20495=DIRECTION ( 'NONE',  ( 0.7066505893342458489, 0.7066505893340067068, 0.03591502732094190020 ) ) ;
#20501=CARTESIAN_POINT ( 'NONE',  ( 63.43270131736515083, 147.4839633491013728, -3.451138109367889228 ) ) ;
#20506=CARTESIAN_POINT ( 'NONE',  ( 43.01140435219951996, 119.9070776186055838, 50.00000000000002842 ) ) ;
#20507=CARTESIAN_POINT ( 'NONE',  ( 17.92634965299622252, 143.2997274935095788, 22.91961472066619265 ) ) ;
#20517=CARTESIAN_POINT ( 'NONE',  ( 49.88381083390898851, 92.64041853056629350, -12.86295667411130239 ) ) ;
#20522=CARTESIAN_POINT ( 'NONE',  ( 45.23168579428472924, 95.00401654713870414, 38.70263932541809737 ) ) ;
#20530=CARTESIAN_POINT ( 'NONE',  ( 21.90415124324598750, 92.95514585177724598, 15.07745334355238676 ) ) ;
#20536=CARTESIAN_POINT ( 'NONE',  ( 14.88286428391304561, 100.3963227437532595, 8.410691821786379307 ) ) ;
#20538=CARTESIAN_POINT ( 'NONE',  ( 51.84853669763433004, 93.12814091139611605, 7.061107544354192633 ) ) ;
#20547=CARTESIAN_POINT ( 'NONE',  ( 44.41273964558330789, 85.70220254879866673, -6.708519844216274564 ) ) ;
#20556=CARTESIAN_POINT ( 'NONE',  ( 37.67147452025017174, 147.5968219552084122, -3.296006884014541782 ) ) ;
#20561=EDGE_LOOP ( 'NONE', ( #8853, #18025 ) ) ;
#20566=CARTESIAN_POINT ( 'NONE',  ( 20.91795382191701336, 137.2581800298614212, 10.90446256675174297 ) ) ;
#20579=CARTESIAN_POINT ( 'NONE',  ( 57.25245068215419053, 144.3413351293631877, -3.490753295080526453 ) ) ;
#20584=CARTESIAN_POINT ( 'NONE',  ( 9.345857484954766647, 125.6588058825717837, 10.27205150250232535 ) ) ;
#20585=CARTESIAN_POINT ( 'NONE',  ( 69.85845278386915425, 111.2786852186620621, 13.01367670771671747 ) ) ;
#20589=VECTOR ( 'NONE', #14293, 1000.000000000000000 ) ;
#20595=CARTESIAN_POINT ( 'NONE',  ( 29.11053999216420252, 151.1052802516552163, -16.63225393015772724 ) ) ;
#20606=CARTESIAN_POINT ( 'NONE',  ( 75.87089013534350102, 129.7906142932847331, -2.736556584054479657 ) ) ;
#20612=CARTESIAN_POINT ( 'NONE',  ( 46.79023103138236905, 91.88018867020078062, 6.271112617211819007 ) ) ;
#20623=CARTESIAN_POINT ( 'NONE',  ( 71.20918238807936973, 120.1790618917378879, 12.65642078274776416 ) ) ;
#20629=CARTESIAN_POINT ( 'NONE',  ( 46.31425486152256354, 95.12510261592046845, 30.44250125826514974 ) ) ;
#20637=CARTESIAN_POINT ( 'NONE',  ( 40.68735894681399401, 154.1427111589966898, 9.763412716672732472 ) ) ;
#20642=CARTESIAN_POINT ( 'NONE',  ( 20.22230697948889500, 94.36241449208007737, 1.148710122009321211 ) ) ;
#20644=CARTESIAN_POINT ( 'NONE',  ( 15.96294818963569639, 111.9339314265907745, 8.846935114401974332 ) ) ;
#20652=CARTESIAN_POINT ( 'NONE',  ( 15.75986397150585816, 99.18880659646561071, -5.637120474378671808 ) ) ;
#20670=CARTESIAN_POINT ( 'NONE',  ( 71.13077487245369923, 119.9619191372588034, 6.660813687590150245 ) ) ;
#20687=CARTESIAN_POINT ( 'NONE',  ( 22.89857099655110062, 139.5608133708311982, -4.966967973427480310 ) ) ;
#20693=CARTESIAN_POINT ( 'NONE',  ( 15.39564893635072806, 140.1373336744895255, -4.208549045858890558 ) ) ;
#20694=CARTESIAN_POINT ( 'NONE',  ( 70.03002323795641360, 111.8333997399938511, 5.989792257250448060 ) ) ;
#20705=CARTESIAN_POINT ( 'NONE',  ( 77.15557362092413030, 120.6950048976143250, -0.4420599252208967100 ) ) ;
#20713=CARTESIAN_POINT ( 'NONE',  ( 10.91571581598819662, 131.8149664739095783, 9.482090752819161139 ) ) ;
#20719=CARTESIAN_POINT ( 'NONE',  ( 28.77282558494574971, 95.47244942437217219, 14.00900696324737282 ) ) ;
#20730=CARTESIAN_POINT ( 'NONE',  ( 15.18239976710701100, 124.4615124019231018, 16.34704286353642999 ) ) ;
#20735=CARTESIAN_POINT ( 'NONE',  ( 47.34993709379126159, 95.28571532017744516, 36.71770137080346785 ) ) ;
#20742=CARTESIAN_POINT ( 'NONE',  ( 15.82680954991375621, 98.96776360684994245, 0.3584833779906905771 ) ) ;
#20747=CARTESIAN_POINT ( 'NONE',  ( 48.17517050666977241, 153.7480039124125994, 4.005852979123367241 ) ) ;
#20751=CARTESIAN_POINT ( 'NONE',  ( 63.07923660420441792, 139.7192868340247571, 4.799362114056002326 ) ) ;
#20757=CARTESIAN_POINT ( 'NONE',  ( 57.94507594753278568, 150.7106492751291569, -2.660852849641732298 ) ) ;
#20761=UNCERTAINTY_MEASURE_WITH_UNIT (LENGTH_MEASURE( 1.000000000000000082E-05 ), #14733, 'distance_accuracy_value', 'NONE');
#20769=CARTESIAN_POINT ( 'NONE',  ( 76.81974253126139729, 125.2811442093199616, -1.589308178208348910 ) ) ;
#20775=CARTESIAN_POINT ( 'NONE',  ( 51.06471579629997137, 92.96554497763615643, 8.089385107838625188 ) ) ;
#20777=CARTESIAN_POINT ( 'NONE',  ( 43.01140435219951996, 119.9070776186055838, 8.284271247461942878 ) ) ;
#20793=CARTESIAN_POINT ( 'NONE',  ( 43.17520790721623314, 91.62706341066298421, 13.41396976009479403 ) ) ;
#20800=CARTESIAN_POINT ( 'NONE',  ( 32.31036143884366396, 152.4250368413922274, -10.51794503956956817 ) ) ;
#20801=CARTESIAN_POINT ( 'NONE',  ( 19.52755003174225124, 104.2962547294809070, 15.51356631106660089 ) ) ;
#20813=CARTESIAN_POINT ( 'NONE',  ( 61.89860894053757789, 148.3622700476249463, -1.513601781051955530 ) ) ;
#20820=CARTESIAN_POINT ( 'NONE',  ( 51.15470623622070434, 86.57325545146775880, 6.072769092256255163 ) ) ;
#20826=CARTESIAN_POINT ( 'NONE',  ( 26.22827968769296092, 97.14409021710402214, 14.12817222279094942 ) ) ;
#20827=CARTESIAN_POINT ( 'NONE',  ( 33.01140435219951286, 119.9070776186055838, -35.00000000000000000 ) ) ;
#20838=CARTESIAN_POINT ( 'NONE',  ( 17.65293208513390866, 132.0582047407114885, -3.339186312533837242 ) ) ;
#20851=CARTESIAN_POINT ( 'NONE',  ( 61.62447910614003632, 148.7338836329059859, 10.47761036752830144 ) ) ;
#20859=CARTESIAN_POINT ( 'NONE',  ( 18.57470074671828542, 105.8336742703428257, 1.585105279193314010 ) ) ;
#20866=CARTESIAN_POINT ( 'NONE',  ( 26.28921445626723852, 149.7786157371718616, -3.732453678475698311 ) ) ;
#20877=CARTESIAN_POINT ( 'NONE',  ( 73.32203938827501588, 103.9946350594383517, -0.8753108214479579097 ) ) ;
#20883=CARTESIAN_POINT ( 'NONE',  ( 23.45433402446531446, 147.8217840461813068, -16.84717431919864339 ) ) ;
#20897=PRODUCT_CONTEXT ( 'NONE', #10431, 'mechanical' ) ;
#20901=CARTESIAN_POINT ( 'NONE',  ( 18.74235739206972085, 134.4262906160203386, 8.771002148563594503 ) ) ;
#20906=CARTESIAN_POINT ( 'NONE',  ( 33.01140435219951286, 119.9070776186055838, -19.99999999999998579 ) ) ;
#20908=CARTESIAN_POINT ( 'NONE',  ( 75.10802748102119608, 108.0013139708956800, -8.018167963582932600 ) ) ;
#20909=CARTESIAN_POINT ( 'NONE',  ( 41.83412315030695794, 148.0818998446914634, 10.87053871734362431 ) ) ;
#20921=CARTESIAN_POINT ( 'NONE',  ( 77.09984031027478579, 117.8059907461747429, -7.347010041119995449 ) ) ;
#20924=CARTESIAN_POINT ( 'NONE',  ( 65.27013532398795803, 145.9152199903044504, 11.62486143609835310 ) ) ;
#20931=CARTESIAN_POINT ( 'NONE',  ( 57.78537588620154963, 150.8774031240512272, 3.334753224648476788 ) ) ;
#20936=CARTESIAN_POINT ( 'NONE',  ( 18.01140435219953062, 119.9070776186055838, 50.00000000000002842 ) ) ;
#20938=CARTESIAN_POINT ( 'NONE',  ( 69.40534582624466964, 109.7482951092767678, 5.080680574306066788 ) ) ;
#20947=CARTESIAN_POINT ( 'NONE',  ( 29.44877014884911404, 144.5398477306827942, -9.648498702473171207 ) ) ;
#20949=CARTESIAN_POINT ( 'NONE',  ( 46.77338793169477782, 144.6226297781437324, 37.50829531803061911 ) ) ;
#20956=CARTESIAN_POINT ( 'NONE',  ( 32.23767430054684979, 145.5917660130465379, 17.43780275515692679 ) ) ;
#20962=CARTESIAN_POINT ( 'NONE',  ( 9.529548018246485341, 127.4200721877477491, 8.334841288026581196 ) ) ;
#20966=EDGE_LOOP ( 'NONE', ( #16095, #10769 ) ) ;
#20968=CARTESIAN_POINT ( 'NONE',  ( 29.12819380265916180, 95.36133955912156068, 0.9897074016940036190 ) ) ;
#20976=CARTESIAN_POINT ( 'NONE',  ( 42.92180000979148957, 85.67454126555050209, 7.339147150375312734 ) ) ;
#20977=CARTESIAN_POINT ( 'NONE',  ( 40.79866406026947345, 95.00477161731822662, 29.72396354041403299 ) ) ;
#20988=CARTESIAN_POINT ( 'NONE',  ( 32.98198692859195802, 152.6383102900375093, -3.493975233523312962 ) ) ;
#20994=CARTESIAN_POINT ( 'NONE',  ( 26.51748177580332566, 149.8140053266110385, -9.728054792207391444 ) ) ;
#21002=CIRCLE ( 'NONE', #17118, 10.00000000000000888 ) ;
#21008=DIRECTION ( 'NONE',  ( 0.000000000000000000, 0.000000000000000000, -1.000000000000000000 ) ) ;
#21015=CARTESIAN_POINT ( 'NONE',  ( 55.65775942066846937, 145.2030105016711445, 10.43785198868815023 ) ) ;
#21021=CARTESIAN_POINT ( 'NONE',  ( 9.468627745026951814, 113.0646104733145592, 1.862908727141013854 ) ) ;
#21022=AXIS2_PLACEMENT_3D ( 'NONE', #14429, #17515, #17839 ) ;
#21023=CARTESIAN_POINT ( 'NONE',  ( 52.77336176550079472, 93.53620953014643646, -12.98192714454240182 ) ) ;
#21033=CARTESIAN_POINT ( 'NONE',  ( 9.953047844039691228, 128.4882722429139505, 3.367556520687803090 ) ) ;
#21034=AXIS2_PLACEMENT_3D ( 'NONE', #12181, #7025, #8675 ) ;
#21038=DIRECTION ( 'NONE',  ( 0.9387810623359078566, 0.3426822732243069436, 0.03548206049944095664 ) ) ;
#21041=CARTESIAN_POINT ( 'NONE',  ( 47.27474595639033339, 153.9548969447091906, 2.977729283044022957 ) ) ;
#21048=CARTESIAN_POINT ( 'NONE',  ( 18.74235739206972085, 134.4262906160203386, 8.771002148563594503 ) ) ;
#21060=CARTESIAN_POINT ( 'NONE',  ( 62.38089001705685632, 99.52138843117178624, -6.434471705120163421 ) ) ;
#21062=CARTESIAN_POINT ( 'NONE',  ( 46.06808526308733320, 144.7210371994902403, 38.18123243450563820 ) ) ;
#21068=CARTESIAN_POINT ( 'NONE',  ( 64.59149290518072917, 93.33317027722591774, -7.422718449586769296 ) ) ;
#21074=CARTESIAN_POINT ( 'NONE',  ( 66.97354912532109950, 95.34500505098478129, 5.477698430975745048 ) ) ;
#21082=CARTESIAN_POINT ( 'NONE',  ( 16.56453993303484395, 129.6948329502664308, 9.561135973024818213 ) ) ;
#21090=CARTESIAN_POINT ( 'NONE',  ( 22.46358530849972723, 92.52609567587644790, 8.053519324161520387 ) ) ;
#21091=CARTESIAN_POINT ( 'NONE',  ( 39.95472344131171383, 95.09311803772094152, 38.18123243450565951 ) ) ;
#21099=CARTESIAN_POINT ( 'NONE',  ( 23.17700876947760591, 147.8092992330439586, -3.851376987104358829 ) ) ;
#21121=CARTESIAN_POINT ( 'NONE',  ( 22.18708823908250238, 100.7722391081675255, 7.342430719951936524 ) ) ;
#21128=CARTESIAN_POINT ( 'NONE',  ( 46.60148787037231699, 85.86292235506145687, 7.220022382731924537 ) ) ;
#21129=CARTESIAN_POINT ( 'NONE',  ( 29.44877014884911404, 144.5398477306827942, -9.648498702473171207 ) ) ;
#21138=CARTESIAN_POINT ( 'NONE',  ( 13.96574040630659752, 137.8735611475157157, -3.299202782472894224 ) ) ;
#21140=CARTESIAN_POINT ( 'NONE',  ( 30.18028515090310293, 151.2280014487710957, 17.43780275515693390 ) ) ;
#21145=CARTESIAN_POINT ( 'NONE',  ( 20.86407471411557779, 93.69780688484533471, 0.1205864258981524662 ) ) ;
#21150=DIRECTION ( 'NONE',  ( -1.186952418100008983E-16, -0.000000000000000000, -1.000000000000000000 ) ) ;
#21152=CARTESIAN_POINT ( 'NONE',  ( 35.68099593698222094, 147.2217917141817907, 16.62841781073025871 ) ) ;
#21162=CARTESIAN_POINT ( 'NONE',  ( 55.45346087869361185, 145.1240540049360845, -8.577242388453932165 ) ) ;
#21164=CARTESIAN_POINT ( 'NONE',  ( 47.35193302267275328, 144.5280796467438620, 36.71405245301005493 ) ) ;
#21169=CARTESIAN_POINT ( 'NONE',  ( 47.47886434171987702, 153.8471147930492862, -3.017879606865911502 ) ) ;
#21175=CARTESIAN_POINT ( 'NONE',  ( 63.63589212299756070, 92.48244826560708987, 12.62055557379543203 ) ) ;
#21184=CIRCLE ( 'NONE', #11669, 3.000000000000050626 ) ;
#21185=CARTESIAN_POINT ( 'NONE',  ( 32.23767430054768823, 145.5917660130458842, 17.43780275515694456 ) ) ;
#21188=CARTESIAN_POINT ( 'NONE',  ( 53.01140435219953417, 119.9070776186055838, -35.00000000000000000 ) ) ;
#21193=CARTESIAN_POINT ( 'NONE',  ( 53.04203944364535772, 87.17698241397053494, 14.00585298808814194 ) ) ;
#21195=CARTESIAN_POINT ( 'NONE',  ( 38.17234397690566539, 95.37979192033441223, 32.91075569967800618 ) ) ;
#21205=CARTESIAN_POINT ( 'NONE',  ( 66.89036333300305159, 144.4373801540182569, -2.303882249869787291 ) ) ;
#21207=AXIS2_PLACEMENT_3D ( 'NONE', #19780, #3023, #21222 ) ;
#21222=DIRECTION ( 'NONE',  ( -0.3428981916074324565, 0.9393725726208703719, 0.000000000000000000 ) ) ;
#21232=CARTESIAN_POINT ( 'NONE',  ( 37.76446383830448639, 92.11682557054228937, 6.628417810721723313 ) ) ;
#21236=VERTEX_POINT ( 'NONE', #11745 ) ;
#21238=CARTESIAN_POINT ( 'NONE',  ( 20.22230697948889500, 94.36241449208007737, 1.148710122009321211 ) ) ;
#21240=CARTESIAN_POINT ( 'NONE',  ( 20.72232308940363765, 137.1362251821529696, 16.90007324815861267 ) ) ;
#21241=CARTESIAN_POINT ( 'NONE',  ( 47.47886434171987702, 153.8471147930492862, -3.017879606865911502 ) ) ;
#21250=CARTESIAN_POINT ( 'NONE',  ( 75.45202302719175691, 109.2280190411066059, 6.938704244663667531 ) ) ;
#21252=CARTESIAN_POINT ( 'NONE',  ( 70.62757080055673953, 99.67629488849819097, 13.29148015538516425 ) ) ;
#21257=CARTESIAN_POINT ( 'NONE',  ( 58.01262221917386341, 89.04620360302797621, 5.834872140203966495 ) ) ;
#21263=CARTESIAN_POINT ( 'NONE',  ( 71.13433436327568415, 121.9840874124550965, -8.414894741535439593 ) ) ;
#21274=CARTESIAN_POINT ( 'NONE',  ( 16.30727314429931241, 128.7156746967485788, -10.48204345529337189 ) ) ;
#21276=CARTESIAN_POINT ( 'NONE',  ( 47.97935898834261081, 144.4085802287884803, 34.86345644064633831 ) ) ;
#21282=CARTESIAN_POINT ( 'NONE',  ( 71.86557814238962294, 101.4853659568252766, -7.779689512009451136 ) ) ;
#21292=CARTESIAN_POINT ( 'NONE',  ( 66.46241511549931147, 94.85692098654722315, 12.50163586956050210 ) ) ;
#21303=CARTESIAN_POINT ( 'NONE',  ( 17.14282613681034917, 97.48634091255654255, 8.291567264837656381 ) ) ;
#21304=CARTESIAN_POINT ( 'NONE',  ( 43.01140435219951996, 94.90707761860558378, 29.21067981925357060 ) ) ;
#21312=CARTESIAN_POINT ( 'NONE',  ( 72.98789752971651978, 103.3738663174133023, 6.148623012889737005 ) ) ;
#21336=CARTESIAN_POINT ( 'NONE',  ( 49.02192908010439254, 147.4586317741252799, -9.843465619175002956 ) ) ;
#21342=CARTESIAN_POINT ( 'NONE',  ( 36.38086904327614235, 86.32171732562966326, 0.5532606071062302622 ) ) ;
#21343=CARTESIAN_POINT ( 'NONE',  ( 43.27907770151751521, 148.0257240122537610, -16.07737750751418915 ) ) ;
#21359=CARTESIAN_POINT ( 'NONE',  ( 25.66908397218059790, 90.29788686741908066, 13.93020729814628744 ) ) ;
#21367=CARTESIAN_POINT ( 'NONE',  ( 60.80507725967250821, 98.03074643439879310, -7.343579217248467295 ) ) ;
#21380=CARTESIAN_POINT ( 'NONE',  ( 15.82502354501850483, 112.7224674592991818, 9.875206726065272278 ) ) ;
#21398=CARTESIAN_POINT ( 'NONE',  ( 12.64719099284060988, 103.9244585094960769, 21.54915782717631600 ) ) ;
#21403=CARTESIAN_POINT ( 'NONE',  ( 36.18411527879869993, 86.44273942418264767, -5.442340506565031433 ) ) ;
#21411=CARTESIAN_POINT ( 'NONE',  ( 70.03002323795641360, 111.8333997399938511, 5.989792257250448060 ) ) ;
#21414=CARTESIAN_POINT ( 'NONE',  ( 75.59501567365037999, 109.4093883240155378, 12.93430809701916750 ) ) ;
#21418=CARTESIAN_POINT ( 'NONE',  ( 41.71434717473703557, 144.8754631261027441, 39.05053369627938054 ) ) ;
#21424=CARTESIAN_POINT ( 'NONE',  ( 47.30009524607925897, 85.94413156685014599, 0.1962900075584997628 ) ) ;
#21447=CARTESIAN_POINT ( 'NONE',  ( 70.54646159239726444, 126.3605644061445901, 18.41388650843374464 ) ) ;
#21453=CARTESIAN_POINT ( 'NONE',  ( 17.60877916486148465, 96.95950790538488206, 1.267834678905774393 ) ) ;
#21454=CARTESIAN_POINT ( 'NONE',  ( 16.34080065753823163, 110.9948608346959276, -11.19624206051981474 ) ) ;
#21472=CARTESIAN_POINT ( 'NONE',  ( 69.75981547520746062, 141.4021063757441823, 10.83457600654633879 ) ) ;
#21481=CARTESIAN_POINT ( 'NONE',  ( 65.38103680468944390, 137.2114283014329317, 17.93782343147312730 ) ) ;
#21492=CARTESIAN_POINT ( 'NONE',  ( 68.61421220432494295, 108.2796574941523886, 7.137043325852385323 ) ) ;
#21503=CARTESIAN_POINT ( 'NONE',  ( 32.14050509837299785, 87.44534670509604268, 7.696117750009315195 ) ) ;
#21507=EDGE_CURVE ( 'NONE', #4221, #460, #14158, .T. ) ;
#21512=CARTESIAN_POINT ( 'NONE',  ( 75.41016232129729246, 131.2110917358880045, 18.21592158385217886 ) ) ;
#21515=CARTESIAN_POINT ( 'NONE',  ( 13.29607544193514990, 103.0715419909171970, -4.489867183945484896 ) ) ;
#21518=CARTESIAN_POINT ( 'NONE',  ( 15.16534570839878349, 115.4582699162533288, 15.98979919289822149 ) ) ;
#21524=CARTESIAN_POINT ( 'NONE',  ( 55.81398226145393693, 145.0329042473489096, 4.442248136324586483 ) ) ;
#21526=CARTESIAN_POINT ( 'NONE',  ( 19.13088699441526686, 95.37848931739559077, 15.19637875606281341 ) ) ;
#21535=CARTESIAN_POINT ( 'NONE',  ( 41.61242760320212852, 154.1118385459532760, 10.79173905232880237 ) ) ;
#21547=AXIS2_PLACEMENT_3D ( 'NONE', #6775, #20214, #3461 ) ;
#21559=CARTESIAN_POINT ( 'NONE',  ( 58.78870511939484800, 143.3781512503299780, 17.58070913143554748 ) ) ;
#21564=CARTESIAN_POINT ( 'NONE',  ( 70.26356658872128946, 140.6255928306487704, 11.86290872716119615 ) ) ;
#21566=CARTESIAN_POINT ( 'NONE',  ( 49.32098446784893753, 92.50438258598539676, -5.839070001793449372 ) ) ;
#21570=ORIENTED_EDGE ( 'NONE', *, *, #19064, .T. ) ;
#21584=CARTESIAN_POINT ( 'NONE',  ( 10.15219960346482431, 110.0225462658725490, 14.76332465322822074 ) ) ;
#21589=CARTESIAN_POINT ( 'NONE',  ( 52.64611633815218283, 152.6728927476294189, 5.153103026933554709 ) ) ;
#21590=CARTESIAN_POINT ( 'NONE',  ( 26.61521700243209310, 142.9206948758876194, 23.22567064538713666 ) ) ;
#21603=CARTESIAN_POINT ( 'NONE',  ( 16.85323768375146614, 130.1535925207217588, 10.57871716905499682 ) ) ;
#21614=CARTESIAN_POINT ( 'NONE',  ( 71.53613896966024299, 138.8348963267899592, -2.065403804986401859 ) ) ;
#21621=CARTESIAN_POINT ( 'NONE',  ( 77.30322022806339533, 121.1324128411339984, 11.54915785461027511 ) ) ;
#21624=CARTESIAN_POINT ( 'NONE',  ( 8.857566569312460558, 119.8222194325741725, -10.91815776494309098 ) ) ;
#21625=EDGE_LOOP ( 'NONE', ( #7929, #14036 ) ) ;
#21634=CARTESIAN_POINT ( 'NONE',  ( 45.98873144221455789, 91.86516812052268222, 7.299390993452533394 ) ) ;
#21642=CARTESIAN_POINT ( 'NONE',  ( 38.01127636974734259, 144.4019489221308277, 33.88560042642480141 ) ) ;
#21647=CARTESIAN_POINT ( 'NONE',  ( 77.22939692449374149, 120.9137088693742044, 5.553548964694690504 ) ) ;
#21654=CARTESIAN_POINT ( 'NONE',  ( 66.89036333300305159, 144.4373801540182569, -2.303882249869787291 ) ) ;
#21662=CARTESIAN_POINT ( 'NONE',  ( 9.345857484954766647, 125.6588058825717837, 10.27205150250232535 ) ) ;
#21672=CARTESIAN_POINT ( 'NONE',  ( 16.98434641657835797, 108.8433182140206270, 14.72356627441054755 ) ) ;
#21678=CARTESIAN_POINT ( 'NONE',  ( 12.61881386508366809, 104.1535352963828984, 15.55354899318430739 ) ) ;
#21680=CARTESIAN_POINT ( 'NONE',  ( 41.47717036631702570, 147.9855288695934803, -2.148757419388624523 ) ) ;
#21695=CARTESIAN_POINT ( 'NONE',  ( 68.49994877969884044, 96.93213776073638144, 19.40600457995573080 ) ) ;
#21699=CARTESIAN_POINT ( 'NONE',  ( 48.37701604703377001, 153.6359454806530778, -1.989754116034292197 ) ) ;
#21700=CARTESIAN_POINT ( 'NONE',  ( 17.48807464456866256, 131.8965856249792523, 2.656420782620954935 ) ) ;
#21703=ORIENTED_EDGE ( 'NONE', *, *, #15831, .T. ) ;
#21711=CARTESIAN_POINT ( 'NONE',  ( 28.48261614285185672, 95.83124311379776827, 2.017784757223194170 ) ) ;
#21715=CARTESIAN_POINT ( 'NONE',  ( 43.01140435219951996, 119.9070776186055838, 50.00000000000002842 ) ) ;
#21721=CARTESIAN_POINT ( 'NONE',  ( 11.39584491653312526, 106.7788786240791978, 8.648593811254444930 ) ) ;
#21728=CARTESIAN_POINT ( 'NONE',  ( 71.19881468907274780, 122.2058620619881566, -2.419290889312981641 ) ) ;
#21731=CARTESIAN_POINT ( 'NONE',  ( 76.67641731516037851, 114.1545672503790740, -7.227887495354823777 ) ) ;
#21740=CARTESIAN_POINT ( 'NONE',  ( 35.91077447413180579, 147.1981228300969633, 10.63281669705329691 ) ) ;
#21743=CARTESIAN_POINT ( 'NONE',  ( 11.08170843061617816, 132.1625483722078513, 16.49545033792581350 ) ) ;
#21747=CARTESIAN_POINT ( 'NONE',  ( 40.79384785287445681, 144.8103769814964608, 29.71740844387221259 ) ) ;
#21752=CARTESIAN_POINT ( 'NONE',  ( 58.57487293839693621, 150.3975950434478648, 4.362879525569486994 ) ) ;
#21763=CARTESIAN_POINT ( 'NONE',  ( 14.94677925004173957, 122.6663546818147381, -4.724578312614759135 ) ) ;
#21770=CARTESIAN_POINT ( 'NONE',  ( 21.78317867943344766, 93.15162560046918827, 9.081842247139665147 ) ) ;
#21771=CARTESIAN_POINT ( 'NONE',  ( 53.01140435219953417, 119.9070776186055838, 8.284271247461942878 ) ) ;
#21780=CARTESIAN_POINT ( 'NONE',  ( 15.11992972970532279, 115.2318815533876375, 21.98540506394948224 ) ) ;
#21786=CARTESIAN_POINT ( 'NONE',  ( 21.43032318156618388, 146.4805633285969861, 10.07716523980869816 ) ) ;
#21788=CARTESIAN_POINT ( 'NONE',  ( 70.89290225163276205, 123.5572941793614206, -0.4820434552990647825 ) ) ;
#21803=CARTESIAN_POINT ( 'NONE',  ( 46.82521527361338087, 85.80558333884177102, 13.21562623509259282 ) ) ;
#21808=CARTESIAN_POINT ( 'NONE',  ( 35.49642027120339094, 86.59030162945495590, 1.581590266896775843 ) ) ;
#21809=CARTESIAN_POINT ( 'NONE',  ( 46.66836841558743032, 147.8683539324387368, -2.938892455568735240 ) ) ;
#21814=DIRECTION ( 'NONE',  ( 1.000000000000000000, 0.000000000000000000, 0.000000000000000000 ) ) ;
ENDSEC;
END-ISO-10303-21;
